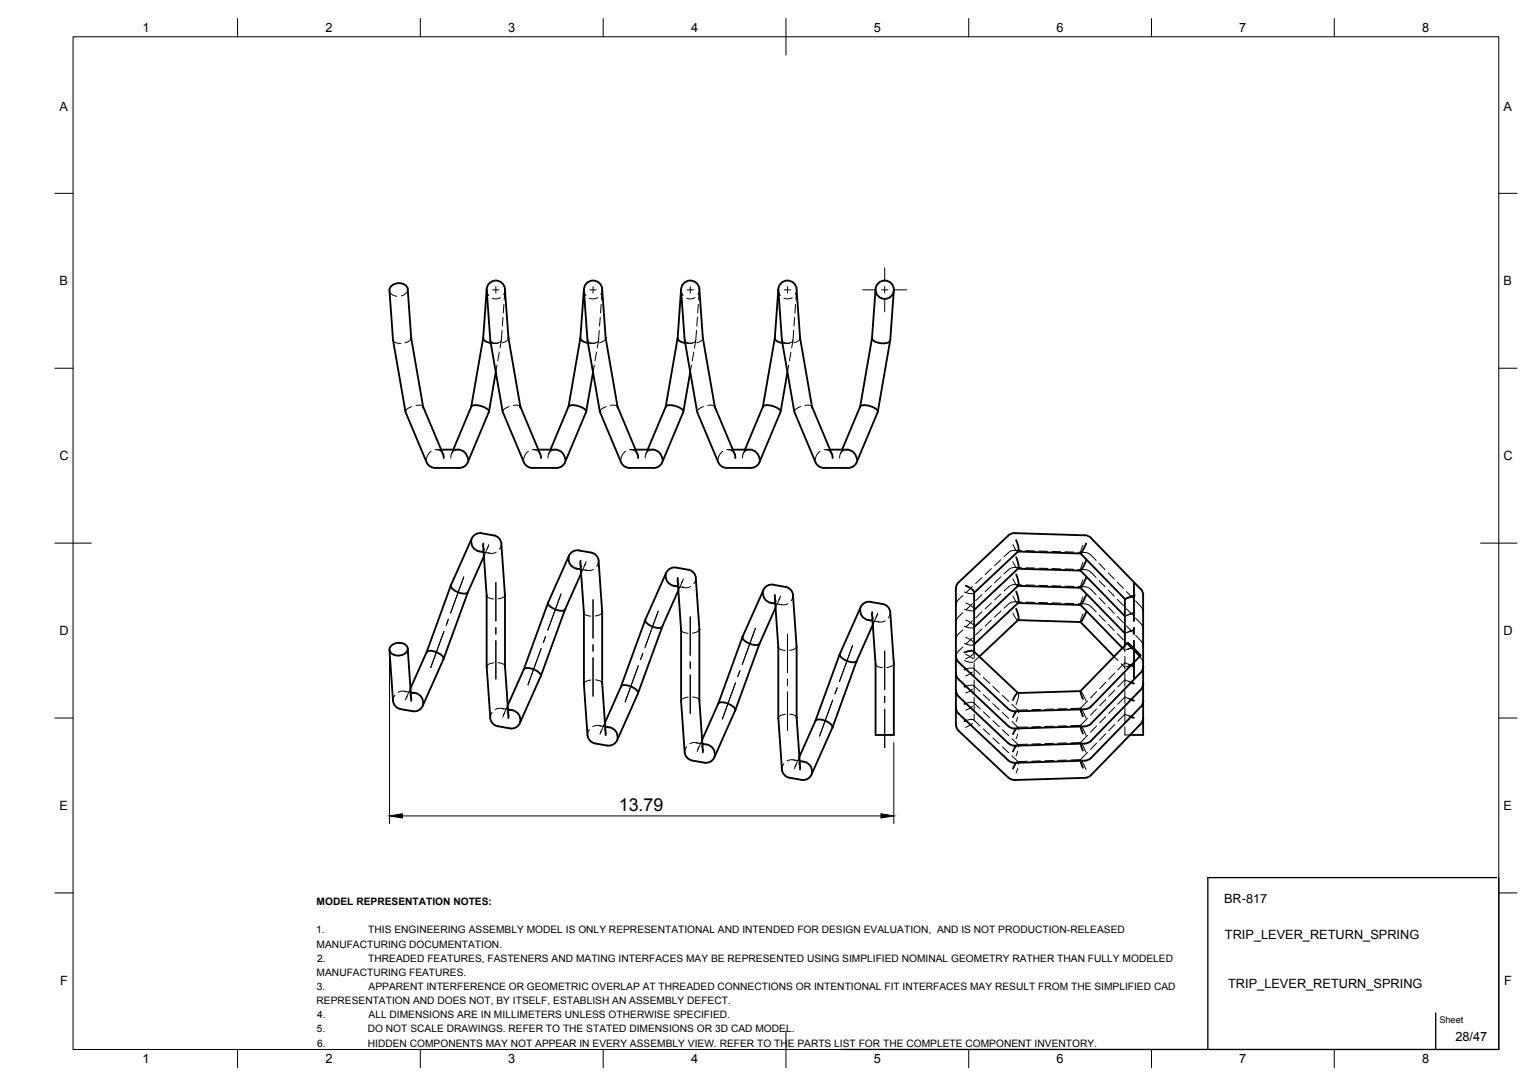
ISO-10303-21;
HEADER;
FILE_DESCRIPTION((''),'2;1');
FILE_NAME('TRIP_LEVER_RETURN_SPRING.step','2026-10-01T22:07:29-07:00',(''),(''),'','','');
FILE_SCHEMA (('AUTOMOTIVE_DESIGN { 1 0 10303 214 3 1 1 }'));
ENDSEC;
DATA;
#10=MECHANICAL_DESIGN_GEOMETRIC_PRESENTATION_REPRESENTATION('',(#560),#15484);
#15=ELLIPSE('',#9204,0.0269900326446259,0.025) ;
#16=ELLIPSE('',#9205,0.0269900326446259,0.025) ;
#17=ELLIPSE('',#9206,0.0269900326446259,0.025) ;
#18=ELLIPSE('',#9209,0.026990032644626,0.025) ;
#19=ELLIPSE('',#9210,0.026990032644626,0.025) ;
#20=ELLIPSE('',#9212,0.026990032644626,0.025) ;
#21=ELLIPSE('',#9214,0.026990032644626,0.025) ;
#22=ELLIPSE('',#9216,0.0269900326446258,0.025) ;
#23=ELLIPSE('',#9218,0.0269900326446259,0.025) ;
#24=ELLIPSE('',#9219,0.0269900326446259,0.025) ;
#25=ELLIPSE('',#9221,0.026990032644626,0.025) ;
#26=ELLIPSE('',#9222,0.026990032644626,0.025) ;
#27=ELLIPSE('',#9223,0.026990032644626,0.025) ;
#28=ELLIPSE('',#9225,0.026990032644626,0.025) ;
#29=ELLIPSE('',#9226,0.026990032644626,0.025) ;
#30=ELLIPSE('',#9228,0.0269900326446259,0.025) ;
#31=ELLIPSE('',#9229,0.0269900326446259,0.025) ;
#32=ELLIPSE('',#9230,0.0269900326446259,0.025) ;
#33=ELLIPSE('',#9232,0.026990032644626,0.025) ;
#34=ELLIPSE('',#9233,0.026990032644626,0.025) ;
#35=ELLIPSE('',#9235,0.0269900326446259,0.025) ;
#36=ELLIPSE('',#9237,0.026990032644626,0.025) ;
#37=ELLIPSE('',#9239,0.026990032644626,0.025) ;
#38=ELLIPSE('',#9241,0.0269900326446259,0.025) ;
#39=ELLIPSE('',#9242,0.0269900326446259,0.025) ;
#40=ELLIPSE('',#9244,0.026990032644626,0.025) ;
#41=ELLIPSE('',#9245,0.026990032644626,0.025) ;
#42=ELLIPSE('',#9246,0.026990032644626,0.025) ;
#43=ELLIPSE('',#9248,0.0269900326446259,0.025) ;
#44=ELLIPSE('',#9249,0.0269900326446259,0.025) ;
#45=ELLIPSE('',#9251,0.0269900326446258,0.025) ;
#46=ELLIPSE('',#9252,0.0269900326446258,0.025) ;
#47=ELLIPSE('',#9253,0.0269900326446258,0.025) ;
#48=ELLIPSE('',#9255,0.0269900326446259,0.025) ;
#49=ELLIPSE('',#9256,0.0269900326446259,0.025) ;
#50=ELLIPSE('',#9258,0.0269900326446259,0.025) ;
#51=ELLIPSE('',#9260,0.026990032644626,0.025) ;
#52=ELLIPSE('',#9262,0.0269900326446259,0.025) ;
#53=ELLIPSE('',#9264,0.026990032644626,0.025) ;
#54=ELLIPSE('',#9265,0.026990032644626,0.025) ;
#55=ELLIPSE('',#9267,0.026990032644626,0.025) ;
#56=ELLIPSE('',#9268,0.026990032644626,0.025) ;
#57=ELLIPSE('',#9269,0.026990032644626,0.025) ;
#58=ELLIPSE('',#9271,0.026990032644626,0.025) ;
#59=ELLIPSE('',#9272,0.026990032644626,0.025) ;
#60=ELLIPSE('',#9274,0.0269900326446259,0.025) ;
#61=ELLIPSE('',#9275,0.0269900326446259,0.025) ;
#62=ELLIPSE('',#9276,0.0269900326446259,0.025) ;
#63=ELLIPSE('',#9278,0.0269900326446259,0.025) ;
#64=ELLIPSE('',#9279,0.0269900326446259,0.025) ;
#65=ELLIPSE('',#9281,0.0269900326446259,0.025) ;
#66=ELLIPSE('',#9283,0.026990032644626,0.025) ;
#67=ELLIPSE('',#9285,0.0269900326446259,0.025) ;
#68=ELLIPSE('',#9287,0.0269900326446259,0.025) ;
#69=ELLIPSE('',#9288,0.0269900326446259,0.025) ;
#70=ELLIPSE('',#9290,0.026990032644626,0.025) ;
#71=ELLIPSE('',#9291,0.026990032644626,0.025) ;
#72=ELLIPSE('',#9292,0.026990032644626,0.025) ;
#73=ELLIPSE('',#9294,0.0269900326446259,0.025) ;
#74=ELLIPSE('',#9295,0.0269900326446259,0.025) ;
#75=ELLIPSE('',#9297,0.0269900326446259,0.025) ;
#76=ELLIPSE('',#9298,0.0269900326446259,0.025) ;
#77=ELLIPSE('',#9299,0.0269900326446259,0.025) ;
#78=ELLIPSE('',#9301,0.0269900326446259,0.025) ;
#79=ELLIPSE('',#9302,0.0269900326446259,0.025) ;
#80=ELLIPSE('',#9304,0.0269900326446259,0.025) ;
#81=ELLIPSE('',#9306,0.026990032644626,0.025) ;
#82=ELLIPSE('',#9308,0.0269900326446259,0.025) ;
#83=ELLIPSE('',#9310,0.026990032644626,0.025) ;
#84=ELLIPSE('',#9311,0.026990032644626,0.025) ;
#85=ELLIPSE('',#9313,0.026990032644626,0.025) ;
#86=ELLIPSE('',#9314,0.026990032644626,0.025) ;
#87=ELLIPSE('',#9315,0.026990032644626,0.025) ;
#198=SPHERICAL_SURFACE('',#9045,0.025) ;
#199=SPHERICAL_SURFACE('',#9048,0.025) ;
#200=SPHERICAL_SURFACE('',#9052,0.025) ;
#201=SPHERICAL_SURFACE('',#9057,0.025) ;
#202=SPHERICAL_SURFACE('',#9062,0.025) ;
#203=SPHERICAL_SURFACE('',#9067,0.025) ;
#204=SPHERICAL_SURFACE('',#9071,0.025) ;
#205=SPHERICAL_SURFACE('',#9074,0.025) ;
#206=SPHERICAL_SURFACE('',#9077,0.025) ;
#207=SPHERICAL_SURFACE('',#9080,0.025) ;
#208=SPHERICAL_SURFACE('',#9084,0.025) ;
#209=SPHERICAL_SURFACE('',#9089,0.025) ;
#210=SPHERICAL_SURFACE('',#9094,0.025) ;
#211=SPHERICAL_SURFACE('',#9099,0.025) ;
#212=SPHERICAL_SURFACE('',#9103,0.025) ;
#213=SPHERICAL_SURFACE('',#9106,0.025) ;
#214=SPHERICAL_SURFACE('',#9109,0.025) ;
#215=SPHERICAL_SURFACE('',#9112,0.025) ;
#216=SPHERICAL_SURFACE('',#9116,0.025) ;
#217=SPHERICAL_SURFACE('',#9121,0.025) ;
#218=SPHERICAL_SURFACE('',#9126,0.025) ;
#219=SPHERICAL_SURFACE('',#9131,0.025) ;
#220=SPHERICAL_SURFACE('',#9135,0.025) ;
#221=SPHERICAL_SURFACE('',#9138,0.025) ;
#222=SPHERICAL_SURFACE('',#9141,0.025) ;
#223=SPHERICAL_SURFACE('',#9144,0.025) ;
#224=SPHERICAL_SURFACE('',#9148,0.025) ;
#225=SPHERICAL_SURFACE('',#9153,0.025) ;
#226=SPHERICAL_SURFACE('',#9158,0.025) ;
#227=SPHERICAL_SURFACE('',#9163,0.025) ;
#228=SPHERICAL_SURFACE('',#9167,0.025) ;
#229=SPHERICAL_SURFACE('',#9170,0.025) ;
#230=SPHERICAL_SURFACE('',#9173,0.025) ;
#231=SPHERICAL_SURFACE('',#9176,0.025) ;
#232=SPHERICAL_SURFACE('',#9180,0.025) ;
#233=SPHERICAL_SURFACE('',#9185,0.025) ;
#234=SPHERICAL_SURFACE('',#9190,0.025) ;
#235=SPHERICAL_SURFACE('',#9195,0.025) ;
#236=SPHERICAL_SURFACE('',#9199,0.025) ;
#490=SHAPE_REPRESENTATION_RELATIONSHIP('SRR','None',#15640,#525) ;
#525=ADVANCED_BREP_SHAPE_REPRESENTATION('',(#601),#15464) ;
#560=STYLED_ITEM('',(#15832),#601) ;
#601=MANIFOLD_SOLID_BREP('TRIP_LEVER_RETURN_SPRING',#8271) ;
#688=CYLINDRICAL_SURFACE('',#9202,0.025) ;
#689=CYLINDRICAL_SURFACE('',#9208,0.025) ;
#690=CYLINDRICAL_SURFACE('',#9211,0.025) ;
#691=CYLINDRICAL_SURFACE('',#9213,0.025) ;
#692=CYLINDRICAL_SURFACE('',#9215,0.025) ;
#693=CYLINDRICAL_SURFACE('',#9217,0.025) ;
#694=CYLINDRICAL_SURFACE('',#9220,0.025) ;
#695=CYLINDRICAL_SURFACE('',#9224,0.025) ;
#696=CYLINDRICAL_SURFACE('',#9227,0.025) ;
#697=CYLINDRICAL_SURFACE('',#9231,0.025) ;
#698=CYLINDRICAL_SURFACE('',#9234,0.025) ;
#699=CYLINDRICAL_SURFACE('',#9236,0.025) ;
#700=CYLINDRICAL_SURFACE('',#9238,0.025) ;
#701=CYLINDRICAL_SURFACE('',#9240,0.025) ;
#702=CYLINDRICAL_SURFACE('',#9243,0.025) ;
#703=CYLINDRICAL_SURFACE('',#9247,0.025) ;
#704=CYLINDRICAL_SURFACE('',#9250,0.025) ;
#705=CYLINDRICAL_SURFACE('',#9254,0.025) ;
#706=CYLINDRICAL_SURFACE('',#9257,0.025) ;
#707=CYLINDRICAL_SURFACE('',#9259,0.025) ;
#708=CYLINDRICAL_SURFACE('',#9261,0.025) ;
#709=CYLINDRICAL_SURFACE('',#9263,0.025) ;
#710=CYLINDRICAL_SURFACE('',#9266,0.025) ;
#711=CYLINDRICAL_SURFACE('',#9270,0.025) ;
#712=CYLINDRICAL_SURFACE('',#9273,0.025) ;
#713=CYLINDRICAL_SURFACE('',#9277,0.025) ;
#714=CYLINDRICAL_SURFACE('',#9280,0.025) ;
#715=CYLINDRICAL_SURFACE('',#9282,0.025) ;
#716=CYLINDRICAL_SURFACE('',#9284,0.025) ;
#717=CYLINDRICAL_SURFACE('',#9286,0.025) ;
#718=CYLINDRICAL_SURFACE('',#9289,0.025) ;
#719=CYLINDRICAL_SURFACE('',#9293,0.025) ;
#720=CYLINDRICAL_SURFACE('',#9296,0.025) ;
#721=CYLINDRICAL_SURFACE('',#9300,0.025) ;
#722=CYLINDRICAL_SURFACE('',#9303,0.025) ;
#723=CYLINDRICAL_SURFACE('',#9305,0.025) ;
#724=CYLINDRICAL_SURFACE('',#9307,0.025) ;
#725=CYLINDRICAL_SURFACE('',#9309,0.025) ;
#726=CYLINDRICAL_SURFACE('',#9312,0.025) ;
#727=CYLINDRICAL_SURFACE('',#9316,0.025) ;
#1019=CIRCLE('',#9046,0.025) ;
#1020=CIRCLE('',#9047,0.025) ;
#1021=CIRCLE('',#9049,0.025) ;
#1022=CIRCLE('',#9050,0.025) ;
#1023=CIRCLE('',#9051,0.025) ;
#1024=CIRCLE('',#9053,0.025) ;
#1025=CIRCLE('',#9054,0.025) ;
#1026=CIRCLE('',#9055,0.025) ;
#1027=CIRCLE('',#9056,0.025) ;
#1028=CIRCLE('',#9058,0.025) ;
#1029=CIRCLE('',#9059,0.025) ;
#1030=CIRCLE('',#9060,0.025) ;
#1031=CIRCLE('',#9061,0.025) ;
#1032=CIRCLE('',#9063,0.025) ;
#1033=CIRCLE('',#9064,0.025) ;
#1034=CIRCLE('',#9065,0.025) ;
#1035=CIRCLE('',#9066,0.025) ;
#1036=CIRCLE('',#9068,0.025) ;
#1037=CIRCLE('',#9069,0.025) ;
#1038=CIRCLE('',#9070,0.025) ;
#1039=CIRCLE('',#9072,0.025) ;
#1040=CIRCLE('',#9073,0.025) ;
#1041=CIRCLE('',#9075,0.025) ;
#1042=CIRCLE('',#9076,0.025) ;
#1043=CIRCLE('',#9078,0.025) ;
#1044=CIRCLE('',#9079,0.025) ;
#1045=CIRCLE('',#9081,0.025) ;
#1046=CIRCLE('',#9082,0.025) ;
#1047=CIRCLE('',#9083,0.025) ;
#1048=CIRCLE('',#9085,0.025) ;
#1049=CIRCLE('',#9086,0.025) ;
#1050=CIRCLE('',#9087,0.025) ;
#1051=CIRCLE('',#9088,0.025) ;
#1052=CIRCLE('',#9090,0.025) ;
#1053=CIRCLE('',#9091,0.025) ;
#1054=CIRCLE('',#9092,0.025) ;
#1055=CIRCLE('',#9093,0.025) ;
#1056=CIRCLE('',#9095,0.025) ;
#1057=CIRCLE('',#9096,0.025) ;
#1058=CIRCLE('',#9097,0.025) ;
#1059=CIRCLE('',#9098,0.025) ;
#1060=CIRCLE('',#9100,0.025) ;
#1061=CIRCLE('',#9101,0.025) ;
#1062=CIRCLE('',#9102,0.025) ;
#1063=CIRCLE('',#9104,0.025) ;
#1064=CIRCLE('',#9105,0.025) ;
#1065=CIRCLE('',#9107,0.025) ;
#1066=CIRCLE('',#9108,0.025) ;
#1067=CIRCLE('',#9110,0.025) ;
#1068=CIRCLE('',#9111,0.025) ;
#1069=CIRCLE('',#9113,0.025) ;
#1070=CIRCLE('',#9114,0.025) ;
#1071=CIRCLE('',#9115,0.025) ;
#1072=CIRCLE('',#9117,0.025) ;
#1073=CIRCLE('',#9118,0.025) ;
#1074=CIRCLE('',#9119,0.025) ;
#1075=CIRCLE('',#9120,0.025) ;
#1076=CIRCLE('',#9122,0.025) ;
#1077=CIRCLE('',#9123,0.025) ;
#1078=CIRCLE('',#9124,0.025) ;
#1079=CIRCLE('',#9125,0.025) ;
#1080=CIRCLE('',#9127,0.025) ;
#1081=CIRCLE('',#9128,0.025) ;
#1082=CIRCLE('',#9129,0.025) ;
#1083=CIRCLE('',#9130,0.025) ;
#1084=CIRCLE('',#9132,0.025) ;
#1085=CIRCLE('',#9133,0.025) ;
#1086=CIRCLE('',#9134,0.025) ;
#1087=CIRCLE('',#9136,0.025) ;
#1088=CIRCLE('',#9137,0.025) ;
#1089=CIRCLE('',#9139,0.025) ;
#1090=CIRCLE('',#9140,0.025) ;
#1091=CIRCLE('',#9142,0.025) ;
#1092=CIRCLE('',#9143,0.025) ;
#1093=CIRCLE('',#9145,0.025) ;
#1094=CIRCLE('',#9146,0.025) ;
#1095=CIRCLE('',#9147,0.025) ;
#1096=CIRCLE('',#9149,0.025) ;
#1097=CIRCLE('',#9150,0.025) ;
#1098=CIRCLE('',#9151,0.025) ;
#1099=CIRCLE('',#9152,0.025) ;
#1100=CIRCLE('',#9154,0.025) ;
#1101=CIRCLE('',#9155,0.025) ;
#1102=CIRCLE('',#9156,0.025) ;
#1103=CIRCLE('',#9157,0.025) ;
#1104=CIRCLE('',#9159,0.025) ;
#1105=CIRCLE('',#9160,0.025) ;
#1106=CIRCLE('',#9161,0.025) ;
#1107=CIRCLE('',#9162,0.025) ;
#1108=CIRCLE('',#9164,0.025) ;
#1109=CIRCLE('',#9165,0.025) ;
#1110=CIRCLE('',#9166,0.025) ;
#1111=CIRCLE('',#9168,0.025) ;
#1112=CIRCLE('',#9169,0.025) ;
#1113=CIRCLE('',#9171,0.025) ;
#1114=CIRCLE('',#9172,0.025) ;
#1115=CIRCLE('',#9174,0.025) ;
#1116=CIRCLE('',#9175,0.025) ;
#1117=CIRCLE('',#9177,0.025) ;
#1118=CIRCLE('',#9178,0.025) ;
#1119=CIRCLE('',#9179,0.025) ;
#1120=CIRCLE('',#9181,0.025) ;
#1121=CIRCLE('',#9182,0.025) ;
#1122=CIRCLE('',#9183,0.025) ;
#1123=CIRCLE('',#9184,0.025) ;
#1124=CIRCLE('',#9186,0.025) ;
#1125=CIRCLE('',#9187,0.025) ;
#1126=CIRCLE('',#9188,0.025) ;
#1127=CIRCLE('',#9189,0.025) ;
#1128=CIRCLE('',#9191,0.025) ;
#1129=CIRCLE('',#9192,0.025) ;
#1130=CIRCLE('',#9193,0.025) ;
#1131=CIRCLE('',#9194,0.025) ;
#1132=CIRCLE('',#9196,0.025) ;
#1133=CIRCLE('',#9197,0.025) ;
#1134=CIRCLE('',#9198,0.025) ;
#1135=CIRCLE('',#9200,0.025) ;
#1136=CIRCLE('',#9201,0.025) ;
#1137=CIRCLE('',#9203,0.025) ;
#1138=CIRCLE('',#9317,0.025) ;
#1554=FACE_OUTER_BOUND('',#2115,.T.) ;
#1555=FACE_OUTER_BOUND('',#2116,.T.) ;
#1556=FACE_OUTER_BOUND('',#2117,.T.) ;
#1557=FACE_OUTER_BOUND('',#2118,.T.) ;
#1558=FACE_OUTER_BOUND('',#2119,.T.) ;
#1559=FACE_OUTER_BOUND('',#2120,.T.) ;
#1560=FACE_OUTER_BOUND('',#2121,.T.) ;
#1561=FACE_OUTER_BOUND('',#2122,.T.) ;
#1562=FACE_OUTER_BOUND('',#2123,.T.) ;
#1563=FACE_OUTER_BOUND('',#2124,.T.) ;
#1564=FACE_OUTER_BOUND('',#2125,.T.) ;
#1565=FACE_OUTER_BOUND('',#2126,.T.) ;
#1566=FACE_OUTER_BOUND('',#2127,.T.) ;
#1567=FACE_OUTER_BOUND('',#2128,.T.) ;
#1568=FACE_OUTER_BOUND('',#2129,.T.) ;
#1569=FACE_OUTER_BOUND('',#2130,.T.) ;
#1570=FACE_OUTER_BOUND('',#2131,.T.) ;
#1571=FACE_OUTER_BOUND('',#2132,.T.) ;
#1572=FACE_OUTER_BOUND('',#2133,.T.) ;
#1573=FACE_OUTER_BOUND('',#2134,.T.) ;
#1574=FACE_OUTER_BOUND('',#2135,.T.) ;
#1575=FACE_OUTER_BOUND('',#2136,.T.) ;
#1576=FACE_OUTER_BOUND('',#2137,.T.) ;
#1577=FACE_OUTER_BOUND('',#2138,.T.) ;
#1578=FACE_OUTER_BOUND('',#2139,.T.) ;
#1579=FACE_OUTER_BOUND('',#2140,.T.) ;
#1580=FACE_OUTER_BOUND('',#2141,.T.) ;
#1581=FACE_OUTER_BOUND('',#2142,.T.) ;
#1582=FACE_OUTER_BOUND('',#2143,.T.) ;
#1583=FACE_OUTER_BOUND('',#2144,.T.) ;
#1584=FACE_OUTER_BOUND('',#2145,.T.) ;
#1585=FACE_OUTER_BOUND('',#2146,.T.) ;
#1586=FACE_OUTER_BOUND('',#2147,.T.) ;
#1587=FACE_OUTER_BOUND('',#2148,.T.) ;
#1588=FACE_OUTER_BOUND('',#2149,.T.) ;
#1589=FACE_OUTER_BOUND('',#2150,.T.) ;
#1590=FACE_OUTER_BOUND('',#2151,.T.) ;
#1591=FACE_OUTER_BOUND('',#2152,.T.) ;
#1592=FACE_OUTER_BOUND('',#2153,.T.) ;
#1593=FACE_OUTER_BOUND('',#2154,.T.) ;
#1594=FACE_OUTER_BOUND('',#2155,.T.) ;
#1595=FACE_OUTER_BOUND('',#2156,.T.) ;
#1596=FACE_OUTER_BOUND('',#2157,.T.) ;
#1597=FACE_OUTER_BOUND('',#2158,.T.) ;
#1598=FACE_OUTER_BOUND('',#2159,.T.) ;
#1599=FACE_OUTER_BOUND('',#2160,.T.) ;
#1600=FACE_OUTER_BOUND('',#2161,.T.) ;
#1601=FACE_OUTER_BOUND('',#2162,.T.) ;
#1602=FACE_OUTER_BOUND('',#2163,.T.) ;
#1603=FACE_OUTER_BOUND('',#2164,.T.) ;
#1604=FACE_OUTER_BOUND('',#2165,.T.) ;
#1605=FACE_OUTER_BOUND('',#2166,.T.) ;
#1606=FACE_OUTER_BOUND('',#2167,.T.) ;
#1607=FACE_OUTER_BOUND('',#2168,.T.) ;
#1608=FACE_OUTER_BOUND('',#2169,.T.) ;
#1609=FACE_OUTER_BOUND('',#2170,.T.) ;
#1610=FACE_OUTER_BOUND('',#2171,.T.) ;
#1611=FACE_OUTER_BOUND('',#2172,.T.) ;
#1612=FACE_OUTER_BOUND('',#2173,.T.) ;
#1613=FACE_OUTER_BOUND('',#2174,.T.) ;
#1614=FACE_OUTER_BOUND('',#2175,.T.) ;
#1615=FACE_OUTER_BOUND('',#2176,.T.) ;
#1616=FACE_OUTER_BOUND('',#2177,.T.) ;
#1617=FACE_OUTER_BOUND('',#2178,.T.) ;
#1618=FACE_OUTER_BOUND('',#2179,.T.) ;
#1619=FACE_OUTER_BOUND('',#2180,.T.) ;
#1620=FACE_OUTER_BOUND('',#2181,.T.) ;
#1621=FACE_OUTER_BOUND('',#2182,.T.) ;
#1622=FACE_OUTER_BOUND('',#2183,.T.) ;
#1623=FACE_OUTER_BOUND('',#2184,.T.) ;
#1624=FACE_OUTER_BOUND('',#2185,.T.) ;
#1625=FACE_OUTER_BOUND('',#2186,.T.) ;
#1626=FACE_OUTER_BOUND('',#2187,.T.) ;
#1627=FACE_OUTER_BOUND('',#2188,.T.) ;
#1628=FACE_OUTER_BOUND('',#2189,.T.) ;
#1629=FACE_OUTER_BOUND('',#2190,.T.) ;
#1630=FACE_OUTER_BOUND('',#2191,.T.) ;
#1631=FACE_OUTER_BOUND('',#2192,.T.) ;
#1632=FACE_OUTER_BOUND('',#2193,.T.) ;
#1633=FACE_OUTER_BOUND('',#2194,.T.) ;
#1634=FACE_OUTER_BOUND('',#2195,.T.) ;
#2115=EDGE_LOOP('',(#6027,#6028)) ;
#2116=EDGE_LOOP('',(#6029,#6030,#6031)) ;
#2117=EDGE_LOOP('',(#6032,#6033,#6034,#6035)) ;
#2118=EDGE_LOOP('',(#6036,#6037,#6038,#6039)) ;
#2119=EDGE_LOOP('',(#6040,#6041,#6042,#6043)) ;
#2120=EDGE_LOOP('',(#6044,#6045,#6046)) ;
#2121=EDGE_LOOP('',(#6047,#6048)) ;
#2122=EDGE_LOOP('',(#6049,#6050)) ;
#2123=EDGE_LOOP('',(#6051,#6052)) ;
#2124=EDGE_LOOP('',(#6053,#6054,#6055)) ;
#2125=EDGE_LOOP('',(#6056,#6057,#6058,#6059)) ;
#2126=EDGE_LOOP('',(#6060,#6061,#6062,#6063)) ;
#2127=EDGE_LOOP('',(#6064,#6065,#6066,#6067)) ;
#2128=EDGE_LOOP('',(#6068,#6069,#6070)) ;
#2129=EDGE_LOOP('',(#6071,#6072)) ;
#2130=EDGE_LOOP('',(#6073,#6074)) ;
#2131=EDGE_LOOP('',(#6075,#6076)) ;
#2132=EDGE_LOOP('',(#6077,#6078,#6079)) ;
#2133=EDGE_LOOP('',(#6080,#6081,#6082,#6083)) ;
#2134=EDGE_LOOP('',(#6084,#6085,#6086,#6087)) ;
#2135=EDGE_LOOP('',(#6088,#6089,#6090,#6091)) ;
#2136=EDGE_LOOP('',(#6092,#6093,#6094)) ;
#2137=EDGE_LOOP('',(#6095,#6096)) ;
#2138=EDGE_LOOP('',(#6097,#6098)) ;
#2139=EDGE_LOOP('',(#6099,#6100)) ;
#2140=EDGE_LOOP('',(#6101,#6102,#6103)) ;
#2141=EDGE_LOOP('',(#6104,#6105,#6106,#6107)) ;
#2142=EDGE_LOOP('',(#6108,#6109,#6110,#6111)) ;
#2143=EDGE_LOOP('',(#6112,#6113,#6114,#6115)) ;
#2144=EDGE_LOOP('',(#6116,#6117,#6118)) ;
#2145=EDGE_LOOP('',(#6119,#6120)) ;
#2146=EDGE_LOOP('',(#6121,#6122)) ;
#2147=EDGE_LOOP('',(#6123,#6124)) ;
#2148=EDGE_LOOP('',(#6125,#6126,#6127)) ;
#2149=EDGE_LOOP('',(#6128,#6129,#6130,#6131)) ;
#2150=EDGE_LOOP('',(#6132,#6133,#6134,#6135)) ;
#2151=EDGE_LOOP('',(#6136,#6137,#6138,#6139)) ;
#2152=EDGE_LOOP('',(#6140,#6141,#6142)) ;
#2153=EDGE_LOOP('',(#6143,#6144)) ;
#2154=EDGE_LOOP('',(#6145,#6146,#6147,#6148,#6149,#6150,#6151)) ;
#2155=EDGE_LOOP('',(#6152)) ;
#2156=EDGE_LOOP('',(#6153,#6154,#6155,#6156,#6157,#6158,#6159,#6160,#6161)) ;
#2157=EDGE_LOOP('',(#6162,#6163,#6164,#6165,#6166,#6167,#6168,#6169,#6170)) ;
#2158=EDGE_LOOP('',(#6171,#6172,#6173,#6174,#6175,#6176,#6177,#6178)) ;
#2159=EDGE_LOOP('',(#6179,#6180,#6181,#6182,#6183,#6184,#6185,#6186)) ;
#2160=EDGE_LOOP('',(#6187,#6188,#6189,#6190,#6191,#6192,#6193,#6194,#6195)) ;
#2161=EDGE_LOOP('',(#6196,#6197,#6198,#6199,#6200,#6201,#6202,#6203,#6204)) ;
#2162=EDGE_LOOP('',(#6205,#6206,#6207,#6208,#6209,#6210,#6211,#6212,#6213)) ;
#2163=EDGE_LOOP('',(#6214,#6215,#6216,#6217,#6218,#6219,#6220,#6221,#6222)) ;
#2164=EDGE_LOOP('',(#6223,#6224,#6225,#6226,#6227,#6228,#6229,#6230,#6231)) ;
#2165=EDGE_LOOP('',(#6232,#6233,#6234,#6235,#6236,#6237,#6238,#6239,#6240)) ;
#2166=EDGE_LOOP('',(#6241,#6242,#6243,#6244,#6245,#6246,#6247,#6248)) ;
#2167=EDGE_LOOP('',(#6249,#6250,#6251,#6252,#6253,#6254,#6255,#6256)) ;
#2168=EDGE_LOOP('',(#6257,#6258,#6259,#6260,#6261,#6262,#6263,#6264,#6265)) ;
#2169=EDGE_LOOP('',(#6266,#6267,#6268,#6269,#6270,#6271,#6272,#6273,#6274)) ;
#2170=EDGE_LOOP('',(#6275,#6276,#6277,#6278,#6279,#6280,#6281,#6282,#6283)) ;
#2171=EDGE_LOOP('',(#6284,#6285,#6286,#6287,#6288,#6289,#6290,#6291,#6292)) ;
#2172=EDGE_LOOP('',(#6293,#6294,#6295,#6296,#6297,#6298,#6299,#6300,#6301)) ;
#2173=EDGE_LOOP('',(#6302,#6303,#6304,#6305,#6306,#6307,#6308,#6309,#6310)) ;
#2174=EDGE_LOOP('',(#6311,#6312,#6313,#6314,#6315,#6316,#6317,#6318)) ;
#2175=EDGE_LOOP('',(#6319,#6320,#6321,#6322,#6323,#6324,#6325,#6326)) ;
#2176=EDGE_LOOP('',(#6327,#6328,#6329,#6330,#6331,#6332,#6333,#6334,#6335)) ;
#2177=EDGE_LOOP('',(#6336,#6337,#6338,#6339,#6340,#6341,#6342,#6343,#6344)) ;
#2178=EDGE_LOOP('',(#6345,#6346,#6347,#6348,#6349,#6350,#6351,#6352,#6353)) ;
#2179=EDGE_LOOP('',(#6354,#6355,#6356,#6357,#6358,#6359,#6360,#6361,#6362)) ;
#2180=EDGE_LOOP('',(#6363,#6364,#6365,#6366,#6367,#6368,#6369,#6370,#6371)) ;
#2181=EDGE_LOOP('',(#6372,#6373,#6374,#6375,#6376,#6377,#6378,#6379,#6380)) ;
#2182=EDGE_LOOP('',(#6381,#6382,#6383,#6384,#6385,#6386,#6387,#6388)) ;
#2183=EDGE_LOOP('',(#6389,#6390,#6391,#6392,#6393,#6394,#6395,#6396)) ;
#2184=EDGE_LOOP('',(#6397,#6398,#6399,#6400,#6401,#6402,#6403,#6404,#6405)) ;
#2185=EDGE_LOOP('',(#6406,#6407,#6408,#6409,#6410,#6411,#6412,#6413,#6414)) ;
#2186=EDGE_LOOP('',(#6415,#6416,#6417,#6418,#6419,#6420,#6421,#6422,#6423)) ;
#2187=EDGE_LOOP('',(#6424,#6425,#6426,#6427,#6428,#6429,#6430,#6431,#6432)) ;
#2188=EDGE_LOOP('',(#6433,#6434,#6435,#6436,#6437,#6438,#6439,#6440,#6441)) ;
#2189=EDGE_LOOP('',(#6442,#6443,#6444,#6445,#6446,#6447,#6448,#6449,#6450)) ;
#2190=EDGE_LOOP('',(#6451,#6452,#6453,#6454,#6455,#6456,#6457,#6458)) ;
#2191=EDGE_LOOP('',(#6459,#6460,#6461,#6462,#6463,#6464,#6465,#6466)) ;
#2192=EDGE_LOOP('',(#6467,#6468,#6469,#6470,#6471,#6472,#6473,#6474,#6475)) ;
#2193=EDGE_LOOP('',(#6476,#6477,#6478,#6479,#6480,#6481,#6482,#6483,#6484)) ;
#2194=EDGE_LOOP('',(#6485,#6486,#6487,#6488,#6489,#6490,#6491)) ;
#2195=EDGE_LOOP('',(#6492)) ;
#2679=LINE('',#14063,#3153) ;
#2680=LINE('',#14071,#3154) ;
#2681=LINE('',#14075,#3155) ;
#2682=LINE('',#14078,#3156) ;
#2683=LINE('',#14081,#3157) ;
#2684=LINE('',#14084,#3158) ;
#2685=LINE('',#14090,#3159) ;
#2686=LINE('',#14097,#3160) ;
#2687=LINE('',#14102,#3161) ;
#2688=LINE('',#14109,#3162) ;
#2689=LINE('',#14113,#3163) ;
#2690=LINE('',#14116,#3164) ;
#2691=LINE('',#14119,#3165) ;
#2692=LINE('',#14122,#3166) ;
#2693=LINE('',#14128,#3167) ;
#2694=LINE('',#14135,#3168) ;
#2695=LINE('',#14140,#3169) ;
#2696=LINE('',#14147,#3170) ;
#2697=LINE('',#14151,#3171) ;
#2698=LINE('',#14154,#3172) ;
#2699=LINE('',#14157,#3173) ;
#2700=LINE('',#14160,#3174) ;
#2701=LINE('',#14166,#3175) ;
#2702=LINE('',#14173,#3176) ;
#2703=LINE('',#14178,#3177) ;
#2704=LINE('',#14185,#3178) ;
#2705=LINE('',#14189,#3179) ;
#2706=LINE('',#14192,#3180) ;
#2707=LINE('',#14195,#3181) ;
#2708=LINE('',#14198,#3182) ;
#2709=LINE('',#14204,#3183) ;
#2710=LINE('',#14211,#3184) ;
#2711=LINE('',#14216,#3185) ;
#2712=LINE('',#14223,#3186) ;
#2713=LINE('',#14227,#3187) ;
#2714=LINE('',#14230,#3188) ;
#2715=LINE('',#14233,#3189) ;
#2716=LINE('',#14236,#3190) ;
#2717=LINE('',#14242,#3191) ;
#2718=LINE('',#14249,#3192) ;
#3153=VECTOR('',#11208,0.025) ;
#3154=VECTOR('',#11219,0.025) ;
#3155=VECTOR('',#11226,0.025) ;
#3156=VECTOR('',#11231,0.025) ;
#3157=VECTOR('',#11236,0.025) ;
#3158=VECTOR('',#11241,0.025) ;
#3159=VECTOR('',#11248,0.025) ;
#3160=VECTOR('',#11257,0.025) ;
#3161=VECTOR('',#11264,0.025) ;
#3162=VECTOR('',#11273,0.025) ;
#3163=VECTOR('',#11280,0.025) ;
#3164=VECTOR('',#11285,0.025) ;
#3165=VECTOR('',#11290,0.025) ;
#3166=VECTOR('',#11295,0.025) ;
#3167=VECTOR('',#11302,0.025) ;
#3168=VECTOR('',#11311,0.025) ;
#3169=VECTOR('',#11318,0.025) ;
#3170=VECTOR('',#11327,0.025) ;
#3171=VECTOR('',#11334,0.025) ;
#3172=VECTOR('',#11339,0.025) ;
#3173=VECTOR('',#11344,0.025) ;
#3174=VECTOR('',#11349,0.025) ;
#3175=VECTOR('',#11356,0.025) ;
#3176=VECTOR('',#11365,0.025) ;
#3177=VECTOR('',#11372,0.025) ;
#3178=VECTOR('',#11381,0.025) ;
#3179=VECTOR('',#11388,0.025) ;
#3180=VECTOR('',#11393,0.025) ;
#3181=VECTOR('',#11398,0.025) ;
#3182=VECTOR('',#11403,0.025) ;
#3183=VECTOR('',#11410,0.025) ;
#3184=VECTOR('',#11419,0.025) ;
#3185=VECTOR('',#11426,0.025) ;
#3186=VECTOR('',#11435,0.025) ;
#3187=VECTOR('',#11442,0.025) ;
#3188=VECTOR('',#11447,0.025) ;
#3189=VECTOR('',#11452,0.025) ;
#3190=VECTOR('',#11457,0.025) ;
#3191=VECTOR('',#11464,0.025) ;
#3192=VECTOR('',#11473,0.025) ;
#3641=VERTEX_POINT('',#13785) ;
#3642=VERTEX_POINT('',#13786) ;
#3643=VERTEX_POINT('',#13790) ;
#3644=VERTEX_POINT('',#13791) ;
#3645=VERTEX_POINT('',#13793) ;
#3646=VERTEX_POINT('',#13797) ;
#3647=VERTEX_POINT('',#13798) ;
#3648=VERTEX_POINT('',#13800) ;
#3649=VERTEX_POINT('',#13802) ;
#3650=VERTEX_POINT('',#13806) ;
#3651=VERTEX_POINT('',#13807) ;
#3652=VERTEX_POINT('',#13809) ;
#3653=VERTEX_POINT('',#13811) ;
#3654=VERTEX_POINT('',#13815) ;
#3655=VERTEX_POINT('',#13816) ;
#3656=VERTEX_POINT('',#13818) ;
#3657=VERTEX_POINT('',#13820) ;
#3658=VERTEX_POINT('',#13824) ;
#3659=VERTEX_POINT('',#13825) ;
#3660=VERTEX_POINT('',#13827) ;
#3661=VERTEX_POINT('',#13831) ;
#3662=VERTEX_POINT('',#13832) ;
#3663=VERTEX_POINT('',#13836) ;
#3664=VERTEX_POINT('',#13837) ;
#3665=VERTEX_POINT('',#13841) ;
#3666=VERTEX_POINT('',#13842) ;
#3667=VERTEX_POINT('',#13846) ;
#3668=VERTEX_POINT('',#13847) ;
#3669=VERTEX_POINT('',#13849) ;
#3670=VERTEX_POINT('',#13853) ;
#3671=VERTEX_POINT('',#13854) ;
#3672=VERTEX_POINT('',#13856) ;
#3673=VERTEX_POINT('',#13858) ;
#3674=VERTEX_POINT('',#13862) ;
#3675=VERTEX_POINT('',#13863) ;
#3676=VERTEX_POINT('',#13865) ;
#3677=VERTEX_POINT('',#13867) ;
#3678=VERTEX_POINT('',#13871) ;
#3679=VERTEX_POINT('',#13872) ;
#3680=VERTEX_POINT('',#13874) ;
#3681=VERTEX_POINT('',#13876) ;
#3682=VERTEX_POINT('',#13880) ;
#3683=VERTEX_POINT('',#13881) ;
#3684=VERTEX_POINT('',#13883) ;
#3685=VERTEX_POINT('',#13887) ;
#3686=VERTEX_POINT('',#13888) ;
#3687=VERTEX_POINT('',#13892) ;
#3688=VERTEX_POINT('',#13893) ;
#3689=VERTEX_POINT('',#13897) ;
#3690=VERTEX_POINT('',#13898) ;
#3691=VERTEX_POINT('',#13902) ;
#3692=VERTEX_POINT('',#13903) ;
#3693=VERTEX_POINT('',#13905) ;
#3694=VERTEX_POINT('',#13909) ;
#3695=VERTEX_POINT('',#13910) ;
#3696=VERTEX_POINT('',#13912) ;
#3697=VERTEX_POINT('',#13914) ;
#3698=VERTEX_POINT('',#13918) ;
#3699=VERTEX_POINT('',#13919) ;
#3700=VERTEX_POINT('',#13921) ;
#3701=VERTEX_POINT('',#13923) ;
#3702=VERTEX_POINT('',#13927) ;
#3703=VERTEX_POINT('',#13928) ;
#3704=VERTEX_POINT('',#13930) ;
#3705=VERTEX_POINT('',#13932) ;
#3706=VERTEX_POINT('',#13936) ;
#3707=VERTEX_POINT('',#13937) ;
#3708=VERTEX_POINT('',#13939) ;
#3709=VERTEX_POINT('',#13943) ;
#3710=VERTEX_POINT('',#13944) ;
#3711=VERTEX_POINT('',#13948) ;
#3712=VERTEX_POINT('',#13949) ;
#3713=VERTEX_POINT('',#13953) ;
#3714=VERTEX_POINT('',#13954) ;
#3715=VERTEX_POINT('',#13958) ;
#3716=VERTEX_POINT('',#13959) ;
#3717=VERTEX_POINT('',#13961) ;
#3718=VERTEX_POINT('',#13965) ;
#3719=VERTEX_POINT('',#13966) ;
#3720=VERTEX_POINT('',#13968) ;
#3721=VERTEX_POINT('',#13970) ;
#3722=VERTEX_POINT('',#13974) ;
#3723=VERTEX_POINT('',#13975) ;
#3724=VERTEX_POINT('',#13977) ;
#3725=VERTEX_POINT('',#13979) ;
#3726=VERTEX_POINT('',#13983) ;
#3727=VERTEX_POINT('',#13984) ;
#3728=VERTEX_POINT('',#13986) ;
#3729=VERTEX_POINT('',#13988) ;
#3730=VERTEX_POINT('',#13992) ;
#3731=VERTEX_POINT('',#13993) ;
#3732=VERTEX_POINT('',#13995) ;
#3733=VERTEX_POINT('',#13999) ;
#3734=VERTEX_POINT('',#14000) ;
#3735=VERTEX_POINT('',#14004) ;
#3736=VERTEX_POINT('',#14005) ;
#3737=VERTEX_POINT('',#14009) ;
#3738=VERTEX_POINT('',#14010) ;
#3739=VERTEX_POINT('',#14014) ;
#3740=VERTEX_POINT('',#14015) ;
#3741=VERTEX_POINT('',#14017) ;
#3742=VERTEX_POINT('',#14021) ;
#3743=VERTEX_POINT('',#14022) ;
#3744=VERTEX_POINT('',#14024) ;
#3745=VERTEX_POINT('',#14026) ;
#3746=VERTEX_POINT('',#14030) ;
#3747=VERTEX_POINT('',#14031) ;
#3748=VERTEX_POINT('',#14033) ;
#3749=VERTEX_POINT('',#14035) ;
#3750=VERTEX_POINT('',#14039) ;
#3751=VERTEX_POINT('',#14040) ;
#3752=VERTEX_POINT('',#14042) ;
#3753=VERTEX_POINT('',#14044) ;
#3754=VERTEX_POINT('',#14048) ;
#3755=VERTEX_POINT('',#14049) ;
#3756=VERTEX_POINT('',#14051) ;
#3757=VERTEX_POINT('',#14055) ;
#3758=VERTEX_POINT('',#14056) ;
#3759=VERTEX_POINT('',#14060) ;
#3760=VERTEX_POINT('',#14062) ;
#3761=VERTEX_POINT('',#14064) ;
#3762=VERTEX_POINT('',#14070) ;
#3763=VERTEX_POINT('',#14085) ;
#3764=VERTEX_POINT('',#14089) ;
#3765=VERTEX_POINT('',#14091) ;
#3766=VERTEX_POINT('',#14096) ;
#3767=VERTEX_POINT('',#14101) ;
#3768=VERTEX_POINT('',#14103) ;
#3769=VERTEX_POINT('',#14108) ;
#3770=VERTEX_POINT('',#14123) ;
#3771=VERTEX_POINT('',#14127) ;
#3772=VERTEX_POINT('',#14129) ;
#3773=VERTEX_POINT('',#14134) ;
#3774=VERTEX_POINT('',#14139) ;
#3775=VERTEX_POINT('',#14141) ;
#3776=VERTEX_POINT('',#14146) ;
#3777=VERTEX_POINT('',#14161) ;
#3778=VERTEX_POINT('',#14165) ;
#3779=VERTEX_POINT('',#14167) ;
#3780=VERTEX_POINT('',#14172) ;
#3781=VERTEX_POINT('',#14177) ;
#3782=VERTEX_POINT('',#14179) ;
#3783=VERTEX_POINT('',#14184) ;
#3784=VERTEX_POINT('',#14199) ;
#3785=VERTEX_POINT('',#14203) ;
#3786=VERTEX_POINT('',#14205) ;
#3787=VERTEX_POINT('',#14210) ;
#3788=VERTEX_POINT('',#14215) ;
#3789=VERTEX_POINT('',#14217) ;
#3790=VERTEX_POINT('',#14222) ;
#3791=VERTEX_POINT('',#14237) ;
#3792=VERTEX_POINT('',#14241) ;
#3793=VERTEX_POINT('',#14243) ;
#3794=VERTEX_POINT('',#14248) ;
#4518=EDGE_CURVE('',#3641,#3642,#1019,.T.) ;
#4519=EDGE_CURVE('',#3642,#3641,#1020,.T.) ;
#4520=EDGE_CURVE('',#3643,#3644,#1021,.T.) ;
#4521=EDGE_CURVE('',#3644,#3645,#1022,.T.) ;
#4522=EDGE_CURVE('',#3645,#3643,#1023,.T.) ;
#4523=EDGE_CURVE('',#3646,#3647,#1024,.T.) ;
#4524=EDGE_CURVE('',#3647,#3648,#1025,.T.) ;
#4525=EDGE_CURVE('',#3648,#3649,#1026,.T.) ;
#4526=EDGE_CURVE('',#3649,#3646,#1027,.T.) ;
#4527=EDGE_CURVE('',#3650,#3651,#1028,.T.) ;
#4528=EDGE_CURVE('',#3651,#3652,#1029,.T.) ;
#4529=EDGE_CURVE('',#3652,#3653,#1030,.T.) ;
#4530=EDGE_CURVE('',#3653,#3650,#1031,.T.) ;
#4531=EDGE_CURVE('',#3654,#3655,#1032,.T.) ;
#4532=EDGE_CURVE('',#3655,#3656,#1033,.T.) ;
#4533=EDGE_CURVE('',#3656,#3657,#1034,.T.) ;
#4534=EDGE_CURVE('',#3657,#3654,#1035,.T.) ;
#4535=EDGE_CURVE('',#3658,#3659,#1036,.T.) ;
#4536=EDGE_CURVE('',#3659,#3660,#1037,.T.) ;
#4537=EDGE_CURVE('',#3660,#3658,#1038,.T.) ;
#4538=EDGE_CURVE('',#3661,#3662,#1039,.T.) ;
#4539=EDGE_CURVE('',#3662,#3661,#1040,.T.) ;
#4540=EDGE_CURVE('',#3663,#3664,#1041,.T.) ;
#4541=EDGE_CURVE('',#3664,#3663,#1042,.T.) ;
#4542=EDGE_CURVE('',#3665,#3666,#1043,.T.) ;
#4543=EDGE_CURVE('',#3666,#3665,#1044,.T.) ;
#4544=EDGE_CURVE('',#3667,#3668,#1045,.T.) ;
#4545=EDGE_CURVE('',#3668,#3669,#1046,.T.) ;
#4546=EDGE_CURVE('',#3669,#3667,#1047,.T.) ;
#4547=EDGE_CURVE('',#3670,#3671,#1048,.T.) ;
#4548=EDGE_CURVE('',#3671,#3672,#1049,.T.) ;
#4549=EDGE_CURVE('',#3672,#3673,#1050,.T.) ;
#4550=EDGE_CURVE('',#3673,#3670,#1051,.T.) ;
#4551=EDGE_CURVE('',#3674,#3675,#1052,.T.) ;
#4552=EDGE_CURVE('',#3675,#3676,#1053,.T.) ;
#4553=EDGE_CURVE('',#3676,#3677,#1054,.T.) ;
#4554=EDGE_CURVE('',#3677,#3674,#1055,.T.) ;
#4555=EDGE_CURVE('',#3678,#3679,#1056,.T.) ;
#4556=EDGE_CURVE('',#3679,#3680,#1057,.T.) ;
#4557=EDGE_CURVE('',#3680,#3681,#1058,.T.) ;
#4558=EDGE_CURVE('',#3681,#3678,#1059,.T.) ;
#4559=EDGE_CURVE('',#3682,#3683,#1060,.T.) ;
#4560=EDGE_CURVE('',#3683,#3684,#1061,.T.) ;
#4561=EDGE_CURVE('',#3684,#3682,#1062,.T.) ;
#4562=EDGE_CURVE('',#3685,#3686,#1063,.T.) ;
#4563=EDGE_CURVE('',#3686,#3685,#1064,.T.) ;
#4564=EDGE_CURVE('',#3687,#3688,#1065,.T.) ;
#4565=EDGE_CURVE('',#3688,#3687,#1066,.T.) ;
#4566=EDGE_CURVE('',#3689,#3690,#1067,.T.) ;
#4567=EDGE_CURVE('',#3690,#3689,#1068,.T.) ;
#4568=EDGE_CURVE('',#3691,#3692,#1069,.T.) ;
#4569=EDGE_CURVE('',#3692,#3693,#1070,.T.) ;
#4570=EDGE_CURVE('',#3693,#3691,#1071,.T.) ;
#4571=EDGE_CURVE('',#3694,#3695,#1072,.T.) ;
#4572=EDGE_CURVE('',#3695,#3696,#1073,.T.) ;
#4573=EDGE_CURVE('',#3696,#3697,#1074,.T.) ;
#4574=EDGE_CURVE('',#3697,#3694,#1075,.T.) ;
#4575=EDGE_CURVE('',#3698,#3699,#1076,.T.) ;
#4576=EDGE_CURVE('',#3699,#3700,#1077,.T.) ;
#4577=EDGE_CURVE('',#3700,#3701,#1078,.T.) ;
#4578=EDGE_CURVE('',#3701,#3698,#1079,.T.) ;
#4579=EDGE_CURVE('',#3702,#3703,#1080,.T.) ;
#4580=EDGE_CURVE('',#3703,#3704,#1081,.T.) ;
#4581=EDGE_CURVE('',#3704,#3705,#1082,.T.) ;
#4582=EDGE_CURVE('',#3705,#3702,#1083,.T.) ;
#4583=EDGE_CURVE('',#3706,#3707,#1084,.T.) ;
#4584=EDGE_CURVE('',#3707,#3708,#1085,.T.) ;
#4585=EDGE_CURVE('',#3708,#3706,#1086,.T.) ;
#4586=EDGE_CURVE('',#3709,#3710,#1087,.T.) ;
#4587=EDGE_CURVE('',#3710,#3709,#1088,.T.) ;
#4588=EDGE_CURVE('',#3711,#3712,#1089,.T.) ;
#4589=EDGE_CURVE('',#3712,#3711,#1090,.T.) ;
#4590=EDGE_CURVE('',#3713,#3714,#1091,.T.) ;
#4591=EDGE_CURVE('',#3714,#3713,#1092,.T.) ;
#4592=EDGE_CURVE('',#3715,#3716,#1093,.T.) ;
#4593=EDGE_CURVE('',#3716,#3717,#1094,.T.) ;
#4594=EDGE_CURVE('',#3717,#3715,#1095,.T.) ;
#4595=EDGE_CURVE('',#3718,#3719,#1096,.T.) ;
#4596=EDGE_CURVE('',#3719,#3720,#1097,.T.) ;
#4597=EDGE_CURVE('',#3720,#3721,#1098,.T.) ;
#4598=EDGE_CURVE('',#3721,#3718,#1099,.T.) ;
#4599=EDGE_CURVE('',#3722,#3723,#1100,.T.) ;
#4600=EDGE_CURVE('',#3723,#3724,#1101,.T.) ;
#4601=EDGE_CURVE('',#3724,#3725,#1102,.T.) ;
#4602=EDGE_CURVE('',#3725,#3722,#1103,.T.) ;
#4603=EDGE_CURVE('',#3726,#3727,#1104,.T.) ;
#4604=EDGE_CURVE('',#3727,#3728,#1105,.T.) ;
#4605=EDGE_CURVE('',#3728,#3729,#1106,.T.) ;
#4606=EDGE_CURVE('',#3729,#3726,#1107,.T.) ;
#4607=EDGE_CURVE('',#3730,#3731,#1108,.T.) ;
#4608=EDGE_CURVE('',#3731,#3732,#1109,.T.) ;
#4609=EDGE_CURVE('',#3732,#3730,#1110,.T.) ;
#4610=EDGE_CURVE('',#3733,#3734,#1111,.T.) ;
#4611=EDGE_CURVE('',#3734,#3733,#1112,.T.) ;
#4612=EDGE_CURVE('',#3735,#3736,#1113,.T.) ;
#4613=EDGE_CURVE('',#3736,#3735,#1114,.T.) ;
#4614=EDGE_CURVE('',#3737,#3738,#1115,.T.) ;
#4615=EDGE_CURVE('',#3738,#3737,#1116,.T.) ;
#4616=EDGE_CURVE('',#3739,#3740,#1117,.T.) ;
#4617=EDGE_CURVE('',#3740,#3741,#1118,.T.) ;
#4618=EDGE_CURVE('',#3741,#3739,#1119,.T.) ;
#4619=EDGE_CURVE('',#3742,#3743,#1120,.T.) ;
#4620=EDGE_CURVE('',#3743,#3744,#1121,.T.) ;
#4621=EDGE_CURVE('',#3744,#3745,#1122,.T.) ;
#4622=EDGE_CURVE('',#3745,#3742,#1123,.T.) ;
#4623=EDGE_CURVE('',#3746,#3747,#1124,.T.) ;
#4624=EDGE_CURVE('',#3747,#3748,#1125,.T.) ;
#4625=EDGE_CURVE('',#3748,#3749,#1126,.T.) ;
#4626=EDGE_CURVE('',#3749,#3746,#1127,.T.) ;
#4627=EDGE_CURVE('',#3750,#3751,#1128,.T.) ;
#4628=EDGE_CURVE('',#3751,#3752,#1129,.T.) ;
#4629=EDGE_CURVE('',#3752,#3753,#1130,.T.) ;
#4630=EDGE_CURVE('',#3753,#3750,#1131,.T.) ;
#4631=EDGE_CURVE('',#3754,#3755,#1132,.T.) ;
#4632=EDGE_CURVE('',#3755,#3756,#1133,.T.) ;
#4633=EDGE_CURVE('',#3756,#3754,#1134,.T.) ;
#4634=EDGE_CURVE('',#3757,#3758,#1135,.T.) ;
#4635=EDGE_CURVE('',#3758,#3757,#1136,.T.) ;
#4636=EDGE_CURVE('',#3759,#3759,#1137,.T.) ;
#4637=EDGE_CURVE('',#3759,#3760,#2679,.T.) ;
#4638=EDGE_CURVE('',#3761,#3760,#15,.T.) ;
#4639=EDGE_CURVE('',#3642,#3761,#16,.T.) ;
#4640=EDGE_CURVE('',#3760,#3641,#17,.T.) ;
#4641=EDGE_CURVE('',#3761,#3762,#2680,.T.) ;
#4642=EDGE_CURVE('',#3644,#3762,#18,.T.) ;
#4643=EDGE_CURVE('',#3762,#3643,#19,.T.) ;
#4644=EDGE_CURVE('',#3645,#3647,#2681,.T.) ;
#4645=EDGE_CURVE('',#3648,#3646,#20,.T.) ;
#4646=EDGE_CURVE('',#3649,#3651,#2682,.T.) ;
#4647=EDGE_CURVE('',#3652,#3650,#21,.T.) ;
#4648=EDGE_CURVE('',#3653,#3655,#2683,.T.) ;
#4649=EDGE_CURVE('',#3656,#3654,#22,.T.) ;
#4650=EDGE_CURVE('',#3657,#3659,#2684,.T.) ;
#4651=EDGE_CURVE('',#3763,#3658,#23,.T.) ;
#4652=EDGE_CURVE('',#3660,#3763,#24,.T.) ;
#4653=EDGE_CURVE('',#3763,#3764,#2685,.T.) ;
#4654=EDGE_CURVE('',#3765,#3764,#25,.T.) ;
#4655=EDGE_CURVE('',#3662,#3765,#26,.T.) ;
#4656=EDGE_CURVE('',#3764,#3661,#27,.T.) ;
#4657=EDGE_CURVE('',#3765,#3766,#2686,.T.) ;
#4658=EDGE_CURVE('',#3664,#3766,#28,.T.) ;
#4659=EDGE_CURVE('',#3766,#3663,#29,.T.) ;
#4660=EDGE_CURVE('',#3766,#3767,#2687,.T.) ;
#4661=EDGE_CURVE('',#3768,#3767,#30,.T.) ;
#4662=EDGE_CURVE('',#3666,#3768,#31,.T.) ;
#4663=EDGE_CURVE('',#3767,#3665,#32,.T.) ;
#4664=EDGE_CURVE('',#3768,#3769,#2688,.T.) ;
#4665=EDGE_CURVE('',#3668,#3769,#33,.T.) ;
#4666=EDGE_CURVE('',#3769,#3667,#34,.T.) ;
#4667=EDGE_CURVE('',#3669,#3671,#2689,.T.) ;
#4668=EDGE_CURVE('',#3672,#3670,#35,.T.) ;
#4669=EDGE_CURVE('',#3673,#3675,#2690,.T.) ;
#4670=EDGE_CURVE('',#3676,#3674,#36,.T.) ;
#4671=EDGE_CURVE('',#3677,#3679,#2691,.T.) ;
#4672=EDGE_CURVE('',#3680,#3678,#37,.T.) ;
#4673=EDGE_CURVE('',#3681,#3683,#2692,.T.) ;
#4674=EDGE_CURVE('',#3770,#3682,#38,.T.) ;
#4675=EDGE_CURVE('',#3684,#3770,#39,.T.) ;
#4676=EDGE_CURVE('',#3770,#3771,#2693,.T.) ;
#4677=EDGE_CURVE('',#3772,#3771,#40,.T.) ;
#4678=EDGE_CURVE('',#3686,#3772,#41,.T.) ;
#4679=EDGE_CURVE('',#3771,#3685,#42,.T.) ;
#4680=EDGE_CURVE('',#3772,#3773,#2694,.T.) ;
#4681=EDGE_CURVE('',#3688,#3773,#43,.T.) ;
#4682=EDGE_CURVE('',#3773,#3687,#44,.T.) ;
#4683=EDGE_CURVE('',#3773,#3774,#2695,.T.) ;
#4684=EDGE_CURVE('',#3775,#3774,#45,.T.) ;
#4685=EDGE_CURVE('',#3690,#3775,#46,.T.) ;
#4686=EDGE_CURVE('',#3774,#3689,#47,.T.) ;
#4687=EDGE_CURVE('',#3775,#3776,#2696,.T.) ;
#4688=EDGE_CURVE('',#3692,#3776,#48,.T.) ;
#4689=EDGE_CURVE('',#3776,#3691,#49,.T.) ;
#4690=EDGE_CURVE('',#3693,#3695,#2697,.T.) ;
#4691=EDGE_CURVE('',#3696,#3694,#50,.T.) ;
#4692=EDGE_CURVE('',#3697,#3699,#2698,.T.) ;
#4693=EDGE_CURVE('',#3700,#3698,#51,.T.) ;
#4694=EDGE_CURVE('',#3701,#3703,#2699,.T.) ;
#4695=EDGE_CURVE('',#3704,#3702,#52,.T.) ;
#4696=EDGE_CURVE('',#3705,#3707,#2700,.T.) ;
#4697=EDGE_CURVE('',#3777,#3706,#53,.T.) ;
#4698=EDGE_CURVE('',#3708,#3777,#54,.T.) ;
#4699=EDGE_CURVE('',#3777,#3778,#2701,.T.) ;
#4700=EDGE_CURVE('',#3779,#3778,#55,.T.) ;
#4701=EDGE_CURVE('',#3710,#3779,#56,.T.) ;
#4702=EDGE_CURVE('',#3778,#3709,#57,.T.) ;
#4703=EDGE_CURVE('',#3779,#3780,#2702,.T.) ;
#4704=EDGE_CURVE('',#3712,#3780,#58,.T.) ;
#4705=EDGE_CURVE('',#3780,#3711,#59,.T.) ;
#4706=EDGE_CURVE('',#3780,#3781,#2703,.T.) ;
#4707=EDGE_CURVE('',#3782,#3781,#60,.T.) ;
#4708=EDGE_CURVE('',#3714,#3782,#61,.T.) ;
#4709=EDGE_CURVE('',#3781,#3713,#62,.T.) ;
#4710=EDGE_CURVE('',#3782,#3783,#2704,.T.) ;
#4711=EDGE_CURVE('',#3716,#3783,#63,.T.) ;
#4712=EDGE_CURVE('',#3783,#3715,#64,.T.) ;
#4713=EDGE_CURVE('',#3717,#3719,#2705,.T.) ;
#4714=EDGE_CURVE('',#3720,#3718,#65,.T.) ;
#4715=EDGE_CURVE('',#3721,#3723,#2706,.T.) ;
#4716=EDGE_CURVE('',#3724,#3722,#66,.T.) ;
#4717=EDGE_CURVE('',#3725,#3727,#2707,.T.) ;
#4718=EDGE_CURVE('',#3728,#3726,#67,.T.) ;
#4719=EDGE_CURVE('',#3729,#3731,#2708,.T.) ;
#4720=EDGE_CURVE('',#3784,#3730,#68,.T.) ;
#4721=EDGE_CURVE('',#3732,#3784,#69,.T.) ;
#4722=EDGE_CURVE('',#3784,#3785,#2709,.T.) ;
#4723=EDGE_CURVE('',#3786,#3785,#70,.T.) ;
#4724=EDGE_CURVE('',#3734,#3786,#71,.T.) ;
#4725=EDGE_CURVE('',#3785,#3733,#72,.T.) ;
#4726=EDGE_CURVE('',#3786,#3787,#2710,.T.) ;
#4727=EDGE_CURVE('',#3736,#3787,#73,.T.) ;
#4728=EDGE_CURVE('',#3787,#3735,#74,.T.) ;
#4729=EDGE_CURVE('',#3787,#3788,#2711,.T.) ;
#4730=EDGE_CURVE('',#3789,#3788,#75,.T.) ;
#4731=EDGE_CURVE('',#3738,#3789,#76,.T.) ;
#4732=EDGE_CURVE('',#3788,#3737,#77,.T.) ;
#4733=EDGE_CURVE('',#3789,#3790,#2712,.T.) ;
#4734=EDGE_CURVE('',#3740,#3790,#78,.T.) ;
#4735=EDGE_CURVE('',#3790,#3739,#79,.T.) ;
#4736=EDGE_CURVE('',#3741,#3743,#2713,.T.) ;
#4737=EDGE_CURVE('',#3744,#3742,#80,.T.) ;
#4738=EDGE_CURVE('',#3745,#3747,#2714,.T.) ;
#4739=EDGE_CURVE('',#3748,#3746,#81,.T.) ;
#4740=EDGE_CURVE('',#3749,#3751,#2715,.T.) ;
#4741=EDGE_CURVE('',#3752,#3750,#82,.T.) ;
#4742=EDGE_CURVE('',#3753,#3755,#2716,.T.) ;
#4743=EDGE_CURVE('',#3791,#3754,#83,.T.) ;
#4744=EDGE_CURVE('',#3756,#3791,#84,.T.) ;
#4745=EDGE_CURVE('',#3791,#3792,#2717,.T.) ;
#4746=EDGE_CURVE('',#3793,#3792,#85,.T.) ;
#4747=EDGE_CURVE('',#3758,#3793,#86,.T.) ;
#4748=EDGE_CURVE('',#3792,#3757,#87,.T.) ;
#4749=EDGE_CURVE('',#3793,#3794,#2718,.T.) ;
#4750=EDGE_CURVE('',#3794,#3794,#1138,.T.) ;
#6027=ORIENTED_EDGE('',*,*,#4518,.T.) ;
#6028=ORIENTED_EDGE('',*,*,#4519,.T.) ;
#6029=ORIENTED_EDGE('',*,*,#4520,.T.) ;
#6030=ORIENTED_EDGE('',*,*,#4521,.T.) ;
#6031=ORIENTED_EDGE('',*,*,#4522,.T.) ;
#6032=ORIENTED_EDGE('',*,*,#4523,.T.) ;
#6033=ORIENTED_EDGE('',*,*,#4524,.T.) ;
#6034=ORIENTED_EDGE('',*,*,#4525,.T.) ;
#6035=ORIENTED_EDGE('',*,*,#4526,.T.) ;
#6036=ORIENTED_EDGE('',*,*,#4527,.T.) ;
#6037=ORIENTED_EDGE('',*,*,#4528,.T.) ;
#6038=ORIENTED_EDGE('',*,*,#4529,.T.) ;
#6039=ORIENTED_EDGE('',*,*,#4530,.T.) ;
#6040=ORIENTED_EDGE('',*,*,#4531,.T.) ;
#6041=ORIENTED_EDGE('',*,*,#4532,.T.) ;
#6042=ORIENTED_EDGE('',*,*,#4533,.T.) ;
#6043=ORIENTED_EDGE('',*,*,#4534,.T.) ;
#6044=ORIENTED_EDGE('',*,*,#4535,.T.) ;
#6045=ORIENTED_EDGE('',*,*,#4536,.T.) ;
#6046=ORIENTED_EDGE('',*,*,#4537,.T.) ;
#6047=ORIENTED_EDGE('',*,*,#4538,.T.) ;
#6048=ORIENTED_EDGE('',*,*,#4539,.T.) ;
#6049=ORIENTED_EDGE('',*,*,#4540,.T.) ;
#6050=ORIENTED_EDGE('',*,*,#4541,.T.) ;
#6051=ORIENTED_EDGE('',*,*,#4542,.T.) ;
#6052=ORIENTED_EDGE('',*,*,#4543,.T.) ;
#6053=ORIENTED_EDGE('',*,*,#4544,.T.) ;
#6054=ORIENTED_EDGE('',*,*,#4545,.T.) ;
#6055=ORIENTED_EDGE('',*,*,#4546,.T.) ;
#6056=ORIENTED_EDGE('',*,*,#4547,.T.) ;
#6057=ORIENTED_EDGE('',*,*,#4548,.T.) ;
#6058=ORIENTED_EDGE('',*,*,#4549,.T.) ;
#6059=ORIENTED_EDGE('',*,*,#4550,.T.) ;
#6060=ORIENTED_EDGE('',*,*,#4551,.T.) ;
#6061=ORIENTED_EDGE('',*,*,#4552,.T.) ;
#6062=ORIENTED_EDGE('',*,*,#4553,.T.) ;
#6063=ORIENTED_EDGE('',*,*,#4554,.T.) ;
#6064=ORIENTED_EDGE('',*,*,#4555,.T.) ;
#6065=ORIENTED_EDGE('',*,*,#4556,.T.) ;
#6066=ORIENTED_EDGE('',*,*,#4557,.T.) ;
#6067=ORIENTED_EDGE('',*,*,#4558,.T.) ;
#6068=ORIENTED_EDGE('',*,*,#4559,.T.) ;
#6069=ORIENTED_EDGE('',*,*,#4560,.T.) ;
#6070=ORIENTED_EDGE('',*,*,#4561,.T.) ;
#6071=ORIENTED_EDGE('',*,*,#4562,.T.) ;
#6072=ORIENTED_EDGE('',*,*,#4563,.T.) ;
#6073=ORIENTED_EDGE('',*,*,#4564,.T.) ;
#6074=ORIENTED_EDGE('',*,*,#4565,.T.) ;
#6075=ORIENTED_EDGE('',*,*,#4566,.T.) ;
#6076=ORIENTED_EDGE('',*,*,#4567,.T.) ;
#6077=ORIENTED_EDGE('',*,*,#4568,.T.) ;
#6078=ORIENTED_EDGE('',*,*,#4569,.T.) ;
#6079=ORIENTED_EDGE('',*,*,#4570,.T.) ;
#6080=ORIENTED_EDGE('',*,*,#4571,.T.) ;
#6081=ORIENTED_EDGE('',*,*,#4572,.T.) ;
#6082=ORIENTED_EDGE('',*,*,#4573,.T.) ;
#6083=ORIENTED_EDGE('',*,*,#4574,.T.) ;
#6084=ORIENTED_EDGE('',*,*,#4575,.T.) ;
#6085=ORIENTED_EDGE('',*,*,#4576,.T.) ;
#6086=ORIENTED_EDGE('',*,*,#4577,.T.) ;
#6087=ORIENTED_EDGE('',*,*,#4578,.T.) ;
#6088=ORIENTED_EDGE('',*,*,#4579,.T.) ;
#6089=ORIENTED_EDGE('',*,*,#4580,.T.) ;
#6090=ORIENTED_EDGE('',*,*,#4581,.T.) ;
#6091=ORIENTED_EDGE('',*,*,#4582,.T.) ;
#6092=ORIENTED_EDGE('',*,*,#4583,.T.) ;
#6093=ORIENTED_EDGE('',*,*,#4584,.T.) ;
#6094=ORIENTED_EDGE('',*,*,#4585,.T.) ;
#6095=ORIENTED_EDGE('',*,*,#4586,.T.) ;
#6096=ORIENTED_EDGE('',*,*,#4587,.T.) ;
#6097=ORIENTED_EDGE('',*,*,#4588,.T.) ;
#6098=ORIENTED_EDGE('',*,*,#4589,.T.) ;
#6099=ORIENTED_EDGE('',*,*,#4590,.T.) ;
#6100=ORIENTED_EDGE('',*,*,#4591,.T.) ;
#6101=ORIENTED_EDGE('',*,*,#4592,.T.) ;
#6102=ORIENTED_EDGE('',*,*,#4593,.T.) ;
#6103=ORIENTED_EDGE('',*,*,#4594,.T.) ;
#6104=ORIENTED_EDGE('',*,*,#4595,.T.) ;
#6105=ORIENTED_EDGE('',*,*,#4596,.T.) ;
#6106=ORIENTED_EDGE('',*,*,#4597,.T.) ;
#6107=ORIENTED_EDGE('',*,*,#4598,.T.) ;
#6108=ORIENTED_EDGE('',*,*,#4599,.T.) ;
#6109=ORIENTED_EDGE('',*,*,#4600,.T.) ;
#6110=ORIENTED_EDGE('',*,*,#4601,.T.) ;
#6111=ORIENTED_EDGE('',*,*,#4602,.T.) ;
#6112=ORIENTED_EDGE('',*,*,#4603,.T.) ;
#6113=ORIENTED_EDGE('',*,*,#4604,.T.) ;
#6114=ORIENTED_EDGE('',*,*,#4605,.T.) ;
#6115=ORIENTED_EDGE('',*,*,#4606,.T.) ;
#6116=ORIENTED_EDGE('',*,*,#4607,.T.) ;
#6117=ORIENTED_EDGE('',*,*,#4608,.T.) ;
#6118=ORIENTED_EDGE('',*,*,#4609,.T.) ;
#6119=ORIENTED_EDGE('',*,*,#4610,.T.) ;
#6120=ORIENTED_EDGE('',*,*,#4611,.T.) ;
#6121=ORIENTED_EDGE('',*,*,#4612,.T.) ;
#6122=ORIENTED_EDGE('',*,*,#4613,.T.) ;
#6123=ORIENTED_EDGE('',*,*,#4614,.T.) ;
#6124=ORIENTED_EDGE('',*,*,#4615,.T.) ;
#6125=ORIENTED_EDGE('',*,*,#4616,.T.) ;
#6126=ORIENTED_EDGE('',*,*,#4617,.T.) ;
#6127=ORIENTED_EDGE('',*,*,#4618,.T.) ;
#6128=ORIENTED_EDGE('',*,*,#4619,.T.) ;
#6129=ORIENTED_EDGE('',*,*,#4620,.T.) ;
#6130=ORIENTED_EDGE('',*,*,#4621,.T.) ;
#6131=ORIENTED_EDGE('',*,*,#4622,.T.) ;
#6132=ORIENTED_EDGE('',*,*,#4623,.T.) ;
#6133=ORIENTED_EDGE('',*,*,#4624,.T.) ;
#6134=ORIENTED_EDGE('',*,*,#4625,.T.) ;
#6135=ORIENTED_EDGE('',*,*,#4626,.T.) ;
#6136=ORIENTED_EDGE('',*,*,#4627,.T.) ;
#6137=ORIENTED_EDGE('',*,*,#4628,.T.) ;
#6138=ORIENTED_EDGE('',*,*,#4629,.T.) ;
#6139=ORIENTED_EDGE('',*,*,#4630,.T.) ;
#6140=ORIENTED_EDGE('',*,*,#4631,.T.) ;
#6141=ORIENTED_EDGE('',*,*,#4632,.T.) ;
#6142=ORIENTED_EDGE('',*,*,#4633,.T.) ;
#6143=ORIENTED_EDGE('',*,*,#4634,.T.) ;
#6144=ORIENTED_EDGE('',*,*,#4635,.T.) ;
#6145=ORIENTED_EDGE('',*,*,#4636,.F.) ;
#6146=ORIENTED_EDGE('',*,*,#4637,.T.) ;
#6147=ORIENTED_EDGE('',*,*,#4638,.F.) ;
#6148=ORIENTED_EDGE('',*,*,#4639,.F.) ;
#6149=ORIENTED_EDGE('',*,*,#4518,.F.) ;
#6150=ORIENTED_EDGE('',*,*,#4640,.F.) ;
#6151=ORIENTED_EDGE('',*,*,#4637,.F.) ;
#6152=ORIENTED_EDGE('',*,*,#4636,.T.) ;
#6153=ORIENTED_EDGE('',*,*,#4639,.T.) ;
#6154=ORIENTED_EDGE('',*,*,#4641,.T.) ;
#6155=ORIENTED_EDGE('',*,*,#4642,.F.) ;
#6156=ORIENTED_EDGE('',*,*,#4520,.F.) ;
#6157=ORIENTED_EDGE('',*,*,#4643,.F.) ;
#6158=ORIENTED_EDGE('',*,*,#4641,.F.) ;
#6159=ORIENTED_EDGE('',*,*,#4638,.T.) ;
#6160=ORIENTED_EDGE('',*,*,#4640,.T.) ;
#6161=ORIENTED_EDGE('',*,*,#4519,.F.) ;
#6162=ORIENTED_EDGE('',*,*,#4642,.T.) ;
#6163=ORIENTED_EDGE('',*,*,#4643,.T.) ;
#6164=ORIENTED_EDGE('',*,*,#4522,.F.) ;
#6165=ORIENTED_EDGE('',*,*,#4644,.T.) ;
#6166=ORIENTED_EDGE('',*,*,#4523,.F.) ;
#6167=ORIENTED_EDGE('',*,*,#4645,.F.) ;
#6168=ORIENTED_EDGE('',*,*,#4524,.F.) ;
#6169=ORIENTED_EDGE('',*,*,#4644,.F.) ;
#6170=ORIENTED_EDGE('',*,*,#4521,.F.) ;
#6171=ORIENTED_EDGE('',*,*,#4645,.T.) ;
#6172=ORIENTED_EDGE('',*,*,#4526,.F.) ;
#6173=ORIENTED_EDGE('',*,*,#4646,.T.) ;
#6174=ORIENTED_EDGE('',*,*,#4527,.F.) ;
#6175=ORIENTED_EDGE('',*,*,#4647,.F.) ;
#6176=ORIENTED_EDGE('',*,*,#4528,.F.) ;
#6177=ORIENTED_EDGE('',*,*,#4646,.F.) ;
#6178=ORIENTED_EDGE('',*,*,#4525,.F.) ;
#6179=ORIENTED_EDGE('',*,*,#4647,.T.) ;
#6180=ORIENTED_EDGE('',*,*,#4530,.F.) ;
#6181=ORIENTED_EDGE('',*,*,#4648,.T.) ;
#6182=ORIENTED_EDGE('',*,*,#4531,.F.) ;
#6183=ORIENTED_EDGE('',*,*,#4649,.F.) ;
#6184=ORIENTED_EDGE('',*,*,#4532,.F.) ;
#6185=ORIENTED_EDGE('',*,*,#4648,.F.) ;
#6186=ORIENTED_EDGE('',*,*,#4529,.F.) ;
#6187=ORIENTED_EDGE('',*,*,#4649,.T.) ;
#6188=ORIENTED_EDGE('',*,*,#4534,.F.) ;
#6189=ORIENTED_EDGE('',*,*,#4650,.T.) ;
#6190=ORIENTED_EDGE('',*,*,#4535,.F.) ;
#6191=ORIENTED_EDGE('',*,*,#4651,.F.) ;
#6192=ORIENTED_EDGE('',*,*,#4652,.F.) ;
#6193=ORIENTED_EDGE('',*,*,#4536,.F.) ;
#6194=ORIENTED_EDGE('',*,*,#4650,.F.) ;
#6195=ORIENTED_EDGE('',*,*,#4533,.F.) ;
#6196=ORIENTED_EDGE('',*,*,#4652,.T.) ;
#6197=ORIENTED_EDGE('',*,*,#4653,.T.) ;
#6198=ORIENTED_EDGE('',*,*,#4654,.F.) ;
#6199=ORIENTED_EDGE('',*,*,#4655,.F.) ;
#6200=ORIENTED_EDGE('',*,*,#4538,.F.) ;
#6201=ORIENTED_EDGE('',*,*,#4656,.F.) ;
#6202=ORIENTED_EDGE('',*,*,#4653,.F.) ;
#6203=ORIENTED_EDGE('',*,*,#4651,.T.) ;
#6204=ORIENTED_EDGE('',*,*,#4537,.F.) ;
#6205=ORIENTED_EDGE('',*,*,#4655,.T.) ;
#6206=ORIENTED_EDGE('',*,*,#4657,.T.) ;
#6207=ORIENTED_EDGE('',*,*,#4658,.F.) ;
#6208=ORIENTED_EDGE('',*,*,#4540,.F.) ;
#6209=ORIENTED_EDGE('',*,*,#4659,.F.) ;
#6210=ORIENTED_EDGE('',*,*,#4657,.F.) ;
#6211=ORIENTED_EDGE('',*,*,#4654,.T.) ;
#6212=ORIENTED_EDGE('',*,*,#4656,.T.) ;
#6213=ORIENTED_EDGE('',*,*,#4539,.F.) ;
#6214=ORIENTED_EDGE('',*,*,#4658,.T.) ;
#6215=ORIENTED_EDGE('',*,*,#4660,.T.) ;
#6216=ORIENTED_EDGE('',*,*,#4661,.F.) ;
#6217=ORIENTED_EDGE('',*,*,#4662,.F.) ;
#6218=ORIENTED_EDGE('',*,*,#4542,.F.) ;
#6219=ORIENTED_EDGE('',*,*,#4663,.F.) ;
#6220=ORIENTED_EDGE('',*,*,#4660,.F.) ;
#6221=ORIENTED_EDGE('',*,*,#4659,.T.) ;
#6222=ORIENTED_EDGE('',*,*,#4541,.F.) ;
#6223=ORIENTED_EDGE('',*,*,#4662,.T.) ;
#6224=ORIENTED_EDGE('',*,*,#4664,.T.) ;
#6225=ORIENTED_EDGE('',*,*,#4665,.F.) ;
#6226=ORIENTED_EDGE('',*,*,#4544,.F.) ;
#6227=ORIENTED_EDGE('',*,*,#4666,.F.) ;
#6228=ORIENTED_EDGE('',*,*,#4664,.F.) ;
#6229=ORIENTED_EDGE('',*,*,#4661,.T.) ;
#6230=ORIENTED_EDGE('',*,*,#4663,.T.) ;
#6231=ORIENTED_EDGE('',*,*,#4543,.F.) ;
#6232=ORIENTED_EDGE('',*,*,#4665,.T.) ;
#6233=ORIENTED_EDGE('',*,*,#4666,.T.) ;
#6234=ORIENTED_EDGE('',*,*,#4546,.F.) ;
#6235=ORIENTED_EDGE('',*,*,#4667,.T.) ;
#6236=ORIENTED_EDGE('',*,*,#4547,.F.) ;
#6237=ORIENTED_EDGE('',*,*,#4668,.F.) ;
#6238=ORIENTED_EDGE('',*,*,#4548,.F.) ;
#6239=ORIENTED_EDGE('',*,*,#4667,.F.) ;
#6240=ORIENTED_EDGE('',*,*,#4545,.F.) ;
#6241=ORIENTED_EDGE('',*,*,#4668,.T.) ;
#6242=ORIENTED_EDGE('',*,*,#4550,.F.) ;
#6243=ORIENTED_EDGE('',*,*,#4669,.T.) ;
#6244=ORIENTED_EDGE('',*,*,#4551,.F.) ;
#6245=ORIENTED_EDGE('',*,*,#4670,.F.) ;
#6246=ORIENTED_EDGE('',*,*,#4552,.F.) ;
#6247=ORIENTED_EDGE('',*,*,#4669,.F.) ;
#6248=ORIENTED_EDGE('',*,*,#4549,.F.) ;
#6249=ORIENTED_EDGE('',*,*,#4670,.T.) ;
#6250=ORIENTED_EDGE('',*,*,#4554,.F.) ;
#6251=ORIENTED_EDGE('',*,*,#4671,.T.) ;
#6252=ORIENTED_EDGE('',*,*,#4555,.F.) ;
#6253=ORIENTED_EDGE('',*,*,#4672,.F.) ;
#6254=ORIENTED_EDGE('',*,*,#4556,.F.) ;
#6255=ORIENTED_EDGE('',*,*,#4671,.F.) ;
#6256=ORIENTED_EDGE('',*,*,#4553,.F.) ;
#6257=ORIENTED_EDGE('',*,*,#4672,.T.) ;
#6258=ORIENTED_EDGE('',*,*,#4558,.F.) ;
#6259=ORIENTED_EDGE('',*,*,#4673,.T.) ;
#6260=ORIENTED_EDGE('',*,*,#4559,.F.) ;
#6261=ORIENTED_EDGE('',*,*,#4674,.F.) ;
#6262=ORIENTED_EDGE('',*,*,#4675,.F.) ;
#6263=ORIENTED_EDGE('',*,*,#4560,.F.) ;
#6264=ORIENTED_EDGE('',*,*,#4673,.F.) ;
#6265=ORIENTED_EDGE('',*,*,#4557,.F.) ;
#6266=ORIENTED_EDGE('',*,*,#4675,.T.) ;
#6267=ORIENTED_EDGE('',*,*,#4676,.T.) ;
#6268=ORIENTED_EDGE('',*,*,#4677,.F.) ;
#6269=ORIENTED_EDGE('',*,*,#4678,.F.) ;
#6270=ORIENTED_EDGE('',*,*,#4562,.F.) ;
#6271=ORIENTED_EDGE('',*,*,#4679,.F.) ;
#6272=ORIENTED_EDGE('',*,*,#4676,.F.) ;
#6273=ORIENTED_EDGE('',*,*,#4674,.T.) ;
#6274=ORIENTED_EDGE('',*,*,#4561,.F.) ;
#6275=ORIENTED_EDGE('',*,*,#4678,.T.) ;
#6276=ORIENTED_EDGE('',*,*,#4680,.T.) ;
#6277=ORIENTED_EDGE('',*,*,#4681,.F.) ;
#6278=ORIENTED_EDGE('',*,*,#4564,.F.) ;
#6279=ORIENTED_EDGE('',*,*,#4682,.F.) ;
#6280=ORIENTED_EDGE('',*,*,#4680,.F.) ;
#6281=ORIENTED_EDGE('',*,*,#4677,.T.) ;
#6282=ORIENTED_EDGE('',*,*,#4679,.T.) ;
#6283=ORIENTED_EDGE('',*,*,#4563,.F.) ;
#6284=ORIENTED_EDGE('',*,*,#4681,.T.) ;
#6285=ORIENTED_EDGE('',*,*,#4683,.T.) ;
#6286=ORIENTED_EDGE('',*,*,#4684,.F.) ;
#6287=ORIENTED_EDGE('',*,*,#4685,.F.) ;
#6288=ORIENTED_EDGE('',*,*,#4566,.F.) ;
#6289=ORIENTED_EDGE('',*,*,#4686,.F.) ;
#6290=ORIENTED_EDGE('',*,*,#4683,.F.) ;
#6291=ORIENTED_EDGE('',*,*,#4682,.T.) ;
#6292=ORIENTED_EDGE('',*,*,#4565,.F.) ;
#6293=ORIENTED_EDGE('',*,*,#4685,.T.) ;
#6294=ORIENTED_EDGE('',*,*,#4687,.T.) ;
#6295=ORIENTED_EDGE('',*,*,#4688,.F.) ;
#6296=ORIENTED_EDGE('',*,*,#4568,.F.) ;
#6297=ORIENTED_EDGE('',*,*,#4689,.F.) ;
#6298=ORIENTED_EDGE('',*,*,#4687,.F.) ;
#6299=ORIENTED_EDGE('',*,*,#4684,.T.) ;
#6300=ORIENTED_EDGE('',*,*,#4686,.T.) ;
#6301=ORIENTED_EDGE('',*,*,#4567,.F.) ;
#6302=ORIENTED_EDGE('',*,*,#4688,.T.) ;
#6303=ORIENTED_EDGE('',*,*,#4689,.T.) ;
#6304=ORIENTED_EDGE('',*,*,#4570,.F.) ;
#6305=ORIENTED_EDGE('',*,*,#4690,.T.) ;
#6306=ORIENTED_EDGE('',*,*,#4571,.F.) ;
#6307=ORIENTED_EDGE('',*,*,#4691,.F.) ;
#6308=ORIENTED_EDGE('',*,*,#4572,.F.) ;
#6309=ORIENTED_EDGE('',*,*,#4690,.F.) ;
#6310=ORIENTED_EDGE('',*,*,#4569,.F.) ;
#6311=ORIENTED_EDGE('',*,*,#4691,.T.) ;
#6312=ORIENTED_EDGE('',*,*,#4574,.F.) ;
#6313=ORIENTED_EDGE('',*,*,#4692,.T.) ;
#6314=ORIENTED_EDGE('',*,*,#4575,.F.) ;
#6315=ORIENTED_EDGE('',*,*,#4693,.F.) ;
#6316=ORIENTED_EDGE('',*,*,#4576,.F.) ;
#6317=ORIENTED_EDGE('',*,*,#4692,.F.) ;
#6318=ORIENTED_EDGE('',*,*,#4573,.F.) ;
#6319=ORIENTED_EDGE('',*,*,#4693,.T.) ;
#6320=ORIENTED_EDGE('',*,*,#4578,.F.) ;
#6321=ORIENTED_EDGE('',*,*,#4694,.T.) ;
#6322=ORIENTED_EDGE('',*,*,#4579,.F.) ;
#6323=ORIENTED_EDGE('',*,*,#4695,.F.) ;
#6324=ORIENTED_EDGE('',*,*,#4580,.F.) ;
#6325=ORIENTED_EDGE('',*,*,#4694,.F.) ;
#6326=ORIENTED_EDGE('',*,*,#4577,.F.) ;
#6327=ORIENTED_EDGE('',*,*,#4695,.T.) ;
#6328=ORIENTED_EDGE('',*,*,#4582,.F.) ;
#6329=ORIENTED_EDGE('',*,*,#4696,.T.) ;
#6330=ORIENTED_EDGE('',*,*,#4583,.F.) ;
#6331=ORIENTED_EDGE('',*,*,#4697,.F.) ;
#6332=ORIENTED_EDGE('',*,*,#4698,.F.) ;
#6333=ORIENTED_EDGE('',*,*,#4584,.F.) ;
#6334=ORIENTED_EDGE('',*,*,#4696,.F.) ;
#6335=ORIENTED_EDGE('',*,*,#4581,.F.) ;
#6336=ORIENTED_EDGE('',*,*,#4698,.T.) ;
#6337=ORIENTED_EDGE('',*,*,#4699,.T.) ;
#6338=ORIENTED_EDGE('',*,*,#4700,.F.) ;
#6339=ORIENTED_EDGE('',*,*,#4701,.F.) ;
#6340=ORIENTED_EDGE('',*,*,#4586,.F.) ;
#6341=ORIENTED_EDGE('',*,*,#4702,.F.) ;
#6342=ORIENTED_EDGE('',*,*,#4699,.F.) ;
#6343=ORIENTED_EDGE('',*,*,#4697,.T.) ;
#6344=ORIENTED_EDGE('',*,*,#4585,.F.) ;
#6345=ORIENTED_EDGE('',*,*,#4701,.T.) ;
#6346=ORIENTED_EDGE('',*,*,#4703,.T.) ;
#6347=ORIENTED_EDGE('',*,*,#4704,.F.) ;
#6348=ORIENTED_EDGE('',*,*,#4588,.F.) ;
#6349=ORIENTED_EDGE('',*,*,#4705,.F.) ;
#6350=ORIENTED_EDGE('',*,*,#4703,.F.) ;
#6351=ORIENTED_EDGE('',*,*,#4700,.T.) ;
#6352=ORIENTED_EDGE('',*,*,#4702,.T.) ;
#6353=ORIENTED_EDGE('',*,*,#4587,.F.) ;
#6354=ORIENTED_EDGE('',*,*,#4704,.T.) ;
#6355=ORIENTED_EDGE('',*,*,#4706,.T.) ;
#6356=ORIENTED_EDGE('',*,*,#4707,.F.) ;
#6357=ORIENTED_EDGE('',*,*,#4708,.F.) ;
#6358=ORIENTED_EDGE('',*,*,#4590,.F.) ;
#6359=ORIENTED_EDGE('',*,*,#4709,.F.) ;
#6360=ORIENTED_EDGE('',*,*,#4706,.F.) ;
#6361=ORIENTED_EDGE('',*,*,#4705,.T.) ;
#6362=ORIENTED_EDGE('',*,*,#4589,.F.) ;
#6363=ORIENTED_EDGE('',*,*,#4708,.T.) ;
#6364=ORIENTED_EDGE('',*,*,#4710,.T.) ;
#6365=ORIENTED_EDGE('',*,*,#4711,.F.) ;
#6366=ORIENTED_EDGE('',*,*,#4592,.F.) ;
#6367=ORIENTED_EDGE('',*,*,#4712,.F.) ;
#6368=ORIENTED_EDGE('',*,*,#4710,.F.) ;
#6369=ORIENTED_EDGE('',*,*,#4707,.T.) ;
#6370=ORIENTED_EDGE('',*,*,#4709,.T.) ;
#6371=ORIENTED_EDGE('',*,*,#4591,.F.) ;
#6372=ORIENTED_EDGE('',*,*,#4711,.T.) ;
#6373=ORIENTED_EDGE('',*,*,#4712,.T.) ;
#6374=ORIENTED_EDGE('',*,*,#4594,.F.) ;
#6375=ORIENTED_EDGE('',*,*,#4713,.T.) ;
#6376=ORIENTED_EDGE('',*,*,#4595,.F.) ;
#6377=ORIENTED_EDGE('',*,*,#4714,.F.) ;
#6378=ORIENTED_EDGE('',*,*,#4596,.F.) ;
#6379=ORIENTED_EDGE('',*,*,#4713,.F.) ;
#6380=ORIENTED_EDGE('',*,*,#4593,.F.) ;
#6381=ORIENTED_EDGE('',*,*,#4714,.T.) ;
#6382=ORIENTED_EDGE('',*,*,#4598,.F.) ;
#6383=ORIENTED_EDGE('',*,*,#4715,.T.) ;
#6384=ORIENTED_EDGE('',*,*,#4599,.F.) ;
#6385=ORIENTED_EDGE('',*,*,#4716,.F.) ;
#6386=ORIENTED_EDGE('',*,*,#4600,.F.) ;
#6387=ORIENTED_EDGE('',*,*,#4715,.F.) ;
#6388=ORIENTED_EDGE('',*,*,#4597,.F.) ;
#6389=ORIENTED_EDGE('',*,*,#4716,.T.) ;
#6390=ORIENTED_EDGE('',*,*,#4602,.F.) ;
#6391=ORIENTED_EDGE('',*,*,#4717,.T.) ;
#6392=ORIENTED_EDGE('',*,*,#4603,.F.) ;
#6393=ORIENTED_EDGE('',*,*,#4718,.F.) ;
#6394=ORIENTED_EDGE('',*,*,#4604,.F.) ;
#6395=ORIENTED_EDGE('',*,*,#4717,.F.) ;
#6396=ORIENTED_EDGE('',*,*,#4601,.F.) ;
#6397=ORIENTED_EDGE('',*,*,#4718,.T.) ;
#6398=ORIENTED_EDGE('',*,*,#4606,.F.) ;
#6399=ORIENTED_EDGE('',*,*,#4719,.T.) ;
#6400=ORIENTED_EDGE('',*,*,#4607,.F.) ;
#6401=ORIENTED_EDGE('',*,*,#4720,.F.) ;
#6402=ORIENTED_EDGE('',*,*,#4721,.F.) ;
#6403=ORIENTED_EDGE('',*,*,#4608,.F.) ;
#6404=ORIENTED_EDGE('',*,*,#4719,.F.) ;
#6405=ORIENTED_EDGE('',*,*,#4605,.F.) ;
#6406=ORIENTED_EDGE('',*,*,#4721,.T.) ;
#6407=ORIENTED_EDGE('',*,*,#4722,.T.) ;
#6408=ORIENTED_EDGE('',*,*,#4723,.F.) ;
#6409=ORIENTED_EDGE('',*,*,#4724,.F.) ;
#6410=ORIENTED_EDGE('',*,*,#4610,.F.) ;
#6411=ORIENTED_EDGE('',*,*,#4725,.F.) ;
#6412=ORIENTED_EDGE('',*,*,#4722,.F.) ;
#6413=ORIENTED_EDGE('',*,*,#4720,.T.) ;
#6414=ORIENTED_EDGE('',*,*,#4609,.F.) ;
#6415=ORIENTED_EDGE('',*,*,#4724,.T.) ;
#6416=ORIENTED_EDGE('',*,*,#4726,.T.) ;
#6417=ORIENTED_EDGE('',*,*,#4727,.F.) ;
#6418=ORIENTED_EDGE('',*,*,#4612,.F.) ;
#6419=ORIENTED_EDGE('',*,*,#4728,.F.) ;
#6420=ORIENTED_EDGE('',*,*,#4726,.F.) ;
#6421=ORIENTED_EDGE('',*,*,#4723,.T.) ;
#6422=ORIENTED_EDGE('',*,*,#4725,.T.) ;
#6423=ORIENTED_EDGE('',*,*,#4611,.F.) ;
#6424=ORIENTED_EDGE('',*,*,#4727,.T.) ;
#6425=ORIENTED_EDGE('',*,*,#4729,.T.) ;
#6426=ORIENTED_EDGE('',*,*,#4730,.F.) ;
#6427=ORIENTED_EDGE('',*,*,#4731,.F.) ;
#6428=ORIENTED_EDGE('',*,*,#4614,.F.) ;
#6429=ORIENTED_EDGE('',*,*,#4732,.F.) ;
#6430=ORIENTED_EDGE('',*,*,#4729,.F.) ;
#6431=ORIENTED_EDGE('',*,*,#4728,.T.) ;
#6432=ORIENTED_EDGE('',*,*,#4613,.F.) ;
#6433=ORIENTED_EDGE('',*,*,#4731,.T.) ;
#6434=ORIENTED_EDGE('',*,*,#4733,.T.) ;
#6435=ORIENTED_EDGE('',*,*,#4734,.F.) ;
#6436=ORIENTED_EDGE('',*,*,#4616,.F.) ;
#6437=ORIENTED_EDGE('',*,*,#4735,.F.) ;
#6438=ORIENTED_EDGE('',*,*,#4733,.F.) ;
#6439=ORIENTED_EDGE('',*,*,#4730,.T.) ;
#6440=ORIENTED_EDGE('',*,*,#4732,.T.) ;
#6441=ORIENTED_EDGE('',*,*,#4615,.F.) ;
#6442=ORIENTED_EDGE('',*,*,#4734,.T.) ;
#6443=ORIENTED_EDGE('',*,*,#4735,.T.) ;
#6444=ORIENTED_EDGE('',*,*,#4618,.F.) ;
#6445=ORIENTED_EDGE('',*,*,#4736,.T.) ;
#6446=ORIENTED_EDGE('',*,*,#4619,.F.) ;
#6447=ORIENTED_EDGE('',*,*,#4737,.F.) ;
#6448=ORIENTED_EDGE('',*,*,#4620,.F.) ;
#6449=ORIENTED_EDGE('',*,*,#4736,.F.) ;
#6450=ORIENTED_EDGE('',*,*,#4617,.F.) ;
#6451=ORIENTED_EDGE('',*,*,#4737,.T.) ;
#6452=ORIENTED_EDGE('',*,*,#4622,.F.) ;
#6453=ORIENTED_EDGE('',*,*,#4738,.T.) ;
#6454=ORIENTED_EDGE('',*,*,#4623,.F.) ;
#6455=ORIENTED_EDGE('',*,*,#4739,.F.) ;
#6456=ORIENTED_EDGE('',*,*,#4624,.F.) ;
#6457=ORIENTED_EDGE('',*,*,#4738,.F.) ;
#6458=ORIENTED_EDGE('',*,*,#4621,.F.) ;
#6459=ORIENTED_EDGE('',*,*,#4739,.T.) ;
#6460=ORIENTED_EDGE('',*,*,#4626,.F.) ;
#6461=ORIENTED_EDGE('',*,*,#4740,.T.) ;
#6462=ORIENTED_EDGE('',*,*,#4627,.F.) ;
#6463=ORIENTED_EDGE('',*,*,#4741,.F.) ;
#6464=ORIENTED_EDGE('',*,*,#4628,.F.) ;
#6465=ORIENTED_EDGE('',*,*,#4740,.F.) ;
#6466=ORIENTED_EDGE('',*,*,#4625,.F.) ;
#6467=ORIENTED_EDGE('',*,*,#4741,.T.) ;
#6468=ORIENTED_EDGE('',*,*,#4630,.F.) ;
#6469=ORIENTED_EDGE('',*,*,#4742,.T.) ;
#6470=ORIENTED_EDGE('',*,*,#4631,.F.) ;
#6471=ORIENTED_EDGE('',*,*,#4743,.F.) ;
#6472=ORIENTED_EDGE('',*,*,#4744,.F.) ;
#6473=ORIENTED_EDGE('',*,*,#4632,.F.) ;
#6474=ORIENTED_EDGE('',*,*,#4742,.F.) ;
#6475=ORIENTED_EDGE('',*,*,#4629,.F.) ;
#6476=ORIENTED_EDGE('',*,*,#4744,.T.) ;
#6477=ORIENTED_EDGE('',*,*,#4745,.T.) ;
#6478=ORIENTED_EDGE('',*,*,#4746,.F.) ;
#6479=ORIENTED_EDGE('',*,*,#4747,.F.) ;
#6480=ORIENTED_EDGE('',*,*,#4634,.F.) ;
#6481=ORIENTED_EDGE('',*,*,#4748,.F.) ;
#6482=ORIENTED_EDGE('',*,*,#4745,.F.) ;
#6483=ORIENTED_EDGE('',*,*,#4743,.T.) ;
#6484=ORIENTED_EDGE('',*,*,#4633,.F.) ;
#6485=ORIENTED_EDGE('',*,*,#4747,.T.) ;
#6486=ORIENTED_EDGE('',*,*,#4749,.T.) ;
#6487=ORIENTED_EDGE('',*,*,#4750,.F.) ;
#6488=ORIENTED_EDGE('',*,*,#4749,.F.) ;
#6489=ORIENTED_EDGE('',*,*,#4746,.T.) ;
#6490=ORIENTED_EDGE('',*,*,#4748,.T.) ;
#6491=ORIENTED_EDGE('',*,*,#4635,.F.) ;
#6492=ORIENTED_EDGE('',*,*,#4750,.T.) ;
#7658=PLANE('',#9207) ;
#7659=PLANE('',#9318) ;
#7941=ADVANCED_FACE('',(#1554),#198,.T.) ;
#7942=ADVANCED_FACE('',(#1555),#199,.T.) ;
#7943=ADVANCED_FACE('',(#1556),#200,.T.) ;
#7944=ADVANCED_FACE('',(#1557),#201,.T.) ;
#7945=ADVANCED_FACE('',(#1558),#202,.T.) ;
#7946=ADVANCED_FACE('',(#1559),#203,.T.) ;
#7947=ADVANCED_FACE('',(#1560),#204,.T.) ;
#7948=ADVANCED_FACE('',(#1561),#205,.T.) ;
#7949=ADVANCED_FACE('',(#1562),#206,.T.) ;
#7950=ADVANCED_FACE('',(#1563),#207,.T.) ;
#7951=ADVANCED_FACE('',(#1564),#208,.T.) ;
#7952=ADVANCED_FACE('',(#1565),#209,.T.) ;
#7953=ADVANCED_FACE('',(#1566),#210,.T.) ;
#7954=ADVANCED_FACE('',(#1567),#211,.T.) ;
#7955=ADVANCED_FACE('',(#1568),#212,.T.) ;
#7956=ADVANCED_FACE('',(#1569),#213,.T.) ;
#7957=ADVANCED_FACE('',(#1570),#214,.T.) ;
#7958=ADVANCED_FACE('',(#1571),#215,.T.) ;
#7959=ADVANCED_FACE('',(#1572),#216,.T.) ;
#7960=ADVANCED_FACE('',(#1573),#217,.T.) ;
#7961=ADVANCED_FACE('',(#1574),#218,.T.) ;
#7962=ADVANCED_FACE('',(#1575),#219,.T.) ;
#7963=ADVANCED_FACE('',(#1576),#220,.T.) ;
#7964=ADVANCED_FACE('',(#1577),#221,.T.) ;
#7965=ADVANCED_FACE('',(#1578),#222,.T.) ;
#7966=ADVANCED_FACE('',(#1579),#223,.T.) ;
#7967=ADVANCED_FACE('',(#1580),#224,.T.) ;
#7968=ADVANCED_FACE('',(#1581),#225,.T.) ;
#7969=ADVANCED_FACE('',(#1582),#226,.T.) ;
#7970=ADVANCED_FACE('',(#1583),#227,.T.) ;
#7971=ADVANCED_FACE('',(#1584),#228,.T.) ;
#7972=ADVANCED_FACE('',(#1585),#229,.T.) ;
#7973=ADVANCED_FACE('',(#1586),#230,.T.) ;
#7974=ADVANCED_FACE('',(#1587),#231,.T.) ;
#7975=ADVANCED_FACE('',(#1588),#232,.T.) ;
#7976=ADVANCED_FACE('',(#1589),#233,.T.) ;
#7977=ADVANCED_FACE('',(#1590),#234,.T.) ;
#7978=ADVANCED_FACE('',(#1591),#235,.T.) ;
#7979=ADVANCED_FACE('',(#1592),#236,.T.) ;
#7980=ADVANCED_FACE('',(#1593),#688,.T.) ;
#7981=ADVANCED_FACE('',(#1594),#7658,.T.) ;
#7982=ADVANCED_FACE('',(#1595),#689,.T.) ;
#7983=ADVANCED_FACE('',(#1596),#690,.T.) ;
#7984=ADVANCED_FACE('',(#1597),#691,.T.) ;
#7985=ADVANCED_FACE('',(#1598),#692,.T.) ;
#7986=ADVANCED_FACE('',(#1599),#693,.T.) ;
#7987=ADVANCED_FACE('',(#1600),#694,.T.) ;
#7988=ADVANCED_FACE('',(#1601),#695,.T.) ;
#7989=ADVANCED_FACE('',(#1602),#696,.T.) ;
#7990=ADVANCED_FACE('',(#1603),#697,.T.) ;
#7991=ADVANCED_FACE('',(#1604),#698,.T.) ;
#7992=ADVANCED_FACE('',(#1605),#699,.T.) ;
#7993=ADVANCED_FACE('',(#1606),#700,.T.) ;
#7994=ADVANCED_FACE('',(#1607),#701,.T.) ;
#7995=ADVANCED_FACE('',(#1608),#702,.T.) ;
#7996=ADVANCED_FACE('',(#1609),#703,.T.) ;
#7997=ADVANCED_FACE('',(#1610),#704,.T.) ;
#7998=ADVANCED_FACE('',(#1611),#705,.T.) ;
#7999=ADVANCED_FACE('',(#1612),#706,.T.) ;
#8000=ADVANCED_FACE('',(#1613),#707,.T.) ;
#8001=ADVANCED_FACE('',(#1614),#708,.T.) ;
#8002=ADVANCED_FACE('',(#1615),#709,.T.) ;
#8003=ADVANCED_FACE('',(#1616),#710,.T.) ;
#8004=ADVANCED_FACE('',(#1617),#711,.T.) ;
#8005=ADVANCED_FACE('',(#1618),#712,.T.) ;
#8006=ADVANCED_FACE('',(#1619),#713,.T.) ;
#8007=ADVANCED_FACE('',(#1620),#714,.T.) ;
#8008=ADVANCED_FACE('',(#1621),#715,.T.) ;
#8009=ADVANCED_FACE('',(#1622),#716,.T.) ;
#8010=ADVANCED_FACE('',(#1623),#717,.T.) ;
#8011=ADVANCED_FACE('',(#1624),#718,.T.) ;
#8012=ADVANCED_FACE('',(#1625),#719,.T.) ;
#8013=ADVANCED_FACE('',(#1626),#720,.T.) ;
#8014=ADVANCED_FACE('',(#1627),#721,.T.) ;
#8015=ADVANCED_FACE('',(#1628),#722,.T.) ;
#8016=ADVANCED_FACE('',(#1629),#723,.T.) ;
#8017=ADVANCED_FACE('',(#1630),#724,.T.) ;
#8018=ADVANCED_FACE('',(#1631),#725,.T.) ;
#8019=ADVANCED_FACE('',(#1632),#726,.T.) ;
#8020=ADVANCED_FACE('',(#1633),#727,.T.) ;
#8021=ADVANCED_FACE('',(#1634),#7659,.T.) ;
#8271=CLOSED_SHELL('',(#7941,#7942,#7943,#7944,#7945,#7946,#7947,#7948,
#7949,#7950,#7951,#7952,#7953,#7954,#7955,#7956,#7957,#7958,#7959,#7960,
#7961,#7962,#7963,#7964,#7965,#7966,#7967,#7968,#7969,#7970,#7971,#7972,
#7973,#7974,#7975,#7976,#7977,#7978,#7979,#7980,#7981,#7982,#7983,#7984,
#7985,#7986,#7987,#7988,#7989,#7990,#7991,#7992,#7993,#7994,#7995,#7996,
#7997,#7998,#7999,#8000,#8001,#8002,#8003,#8004,#8005,#8006,#8007,#8008,
#8009,#8010,#8011,#8012,#8013,#8014,#8015,#8016,#8017,#8018,#8019,#8020,
#8021)) ;
#9044=AXIS2_PLACEMENT_3D('',#13783,#10888,#10889) ;
#9045=AXIS2_PLACEMENT_3D('',#13784,#10890,#10891) ;
#9046=AXIS2_PLACEMENT_3D('',#13787,#10892,#10893) ;
#9047=AXIS2_PLACEMENT_3D('',#13788,#10894,#10895) ;
#9048=AXIS2_PLACEMENT_3D('',#13789,#10896,#10897) ;
#9049=AXIS2_PLACEMENT_3D('',#13792,#10898,#10899) ;
#9050=AXIS2_PLACEMENT_3D('',#13794,#10900,#10901) ;
#9051=AXIS2_PLACEMENT_3D('',#13795,#10902,#10903) ;
#9052=AXIS2_PLACEMENT_3D('',#13796,#10904,#10905) ;
#9053=AXIS2_PLACEMENT_3D('',#13799,#10906,#10907) ;
#9054=AXIS2_PLACEMENT_3D('',#13801,#10908,#10909) ;
#9055=AXIS2_PLACEMENT_3D('',#13803,#10910,#10911) ;
#9056=AXIS2_PLACEMENT_3D('',#13804,#10912,#10913) ;
#9057=AXIS2_PLACEMENT_3D('',#13805,#10914,#10915) ;
#9058=AXIS2_PLACEMENT_3D('',#13808,#10916,#10917) ;
#9059=AXIS2_PLACEMENT_3D('',#13810,#10918,#10919) ;
#9060=AXIS2_PLACEMENT_3D('',#13812,#10920,#10921) ;
#9061=AXIS2_PLACEMENT_3D('',#13813,#10922,#10923) ;
#9062=AXIS2_PLACEMENT_3D('',#13814,#10924,#10925) ;
#9063=AXIS2_PLACEMENT_3D('',#13817,#10926,#10927) ;
#9064=AXIS2_PLACEMENT_3D('',#13819,#10928,#10929) ;
#9065=AXIS2_PLACEMENT_3D('',#13821,#10930,#10931) ;
#9066=AXIS2_PLACEMENT_3D('',#13822,#10932,#10933) ;
#9067=AXIS2_PLACEMENT_3D('',#13823,#10934,#10935) ;
#9068=AXIS2_PLACEMENT_3D('',#13826,#10936,#10937) ;
#9069=AXIS2_PLACEMENT_3D('',#13828,#10938,#10939) ;
#9070=AXIS2_PLACEMENT_3D('',#13829,#10940,#10941) ;
#9071=AXIS2_PLACEMENT_3D('',#13830,#10942,#10943) ;
#9072=AXIS2_PLACEMENT_3D('',#13833,#10944,#10945) ;
#9073=AXIS2_PLACEMENT_3D('',#13834,#10946,#10947) ;
#9074=AXIS2_PLACEMENT_3D('',#13835,#10948,#10949) ;
#9075=AXIS2_PLACEMENT_3D('',#13838,#10950,#10951) ;
#9076=AXIS2_PLACEMENT_3D('',#13839,#10952,#10953) ;
#9077=AXIS2_PLACEMENT_3D('',#13840,#10954,#10955) ;
#9078=AXIS2_PLACEMENT_3D('',#13843,#10956,#10957) ;
#9079=AXIS2_PLACEMENT_3D('',#13844,#10958,#10959) ;
#9080=AXIS2_PLACEMENT_3D('',#13845,#10960,#10961) ;
#9081=AXIS2_PLACEMENT_3D('',#13848,#10962,#10963) ;
#9082=AXIS2_PLACEMENT_3D('',#13850,#10964,#10965) ;
#9083=AXIS2_PLACEMENT_3D('',#13851,#10966,#10967) ;
#9084=AXIS2_PLACEMENT_3D('',#13852,#10968,#10969) ;
#9085=AXIS2_PLACEMENT_3D('',#13855,#10970,#10971) ;
#9086=AXIS2_PLACEMENT_3D('',#13857,#10972,#10973) ;
#9087=AXIS2_PLACEMENT_3D('',#13859,#10974,#10975) ;
#9088=AXIS2_PLACEMENT_3D('',#13860,#10976,#10977) ;
#9089=AXIS2_PLACEMENT_3D('',#13861,#10978,#10979) ;
#9090=AXIS2_PLACEMENT_3D('',#13864,#10980,#10981) ;
#9091=AXIS2_PLACEMENT_3D('',#13866,#10982,#10983) ;
#9092=AXIS2_PLACEMENT_3D('',#13868,#10984,#10985) ;
#9093=AXIS2_PLACEMENT_3D('',#13869,#10986,#10987) ;
#9094=AXIS2_PLACEMENT_3D('',#13870,#10988,#10989) ;
#9095=AXIS2_PLACEMENT_3D('',#13873,#10990,#10991) ;
#9096=AXIS2_PLACEMENT_3D('',#13875,#10992,#10993) ;
#9097=AXIS2_PLACEMENT_3D('',#13877,#10994,#10995) ;
#9098=AXIS2_PLACEMENT_3D('',#13878,#10996,#10997) ;
#9099=AXIS2_PLACEMENT_3D('',#13879,#10998,#10999) ;
#9100=AXIS2_PLACEMENT_3D('',#13882,#11000,#11001) ;
#9101=AXIS2_PLACEMENT_3D('',#13884,#11002,#11003) ;
#9102=AXIS2_PLACEMENT_3D('',#13885,#11004,#11005) ;
#9103=AXIS2_PLACEMENT_3D('',#13886,#11006,#11007) ;
#9104=AXIS2_PLACEMENT_3D('',#13889,#11008,#11009) ;
#9105=AXIS2_PLACEMENT_3D('',#13890,#11010,#11011) ;
#9106=AXIS2_PLACEMENT_3D('',#13891,#11012,#11013) ;
#9107=AXIS2_PLACEMENT_3D('',#13894,#11014,#11015) ;
#9108=AXIS2_PLACEMENT_3D('',#13895,#11016,#11017) ;
#9109=AXIS2_PLACEMENT_3D('',#13896,#11018,#11019) ;
#9110=AXIS2_PLACEMENT_3D('',#13899,#11020,#11021) ;
#9111=AXIS2_PLACEMENT_3D('',#13900,#11022,#11023) ;
#9112=AXIS2_PLACEMENT_3D('',#13901,#11024,#11025) ;
#9113=AXIS2_PLACEMENT_3D('',#13904,#11026,#11027) ;
#9114=AXIS2_PLACEMENT_3D('',#13906,#11028,#11029) ;
#9115=AXIS2_PLACEMENT_3D('',#13907,#11030,#11031) ;
#9116=AXIS2_PLACEMENT_3D('',#13908,#11032,#11033) ;
#9117=AXIS2_PLACEMENT_3D('',#13911,#11034,#11035) ;
#9118=AXIS2_PLACEMENT_3D('',#13913,#11036,#11037) ;
#9119=AXIS2_PLACEMENT_3D('',#13915,#11038,#11039) ;
#9120=AXIS2_PLACEMENT_3D('',#13916,#11040,#11041) ;
#9121=AXIS2_PLACEMENT_3D('',#13917,#11042,#11043) ;
#9122=AXIS2_PLACEMENT_3D('',#13920,#11044,#11045) ;
#9123=AXIS2_PLACEMENT_3D('',#13922,#11046,#11047) ;
#9124=AXIS2_PLACEMENT_3D('',#13924,#11048,#11049) ;
#9125=AXIS2_PLACEMENT_3D('',#13925,#11050,#11051) ;
#9126=AXIS2_PLACEMENT_3D('',#13926,#11052,#11053) ;
#9127=AXIS2_PLACEMENT_3D('',#13929,#11054,#11055) ;
#9128=AXIS2_PLACEMENT_3D('',#13931,#11056,#11057) ;
#9129=AXIS2_PLACEMENT_3D('',#13933,#11058,#11059) ;
#9130=AXIS2_PLACEMENT_3D('',#13934,#11060,#11061) ;
#9131=AXIS2_PLACEMENT_3D('',#13935,#11062,#11063) ;
#9132=AXIS2_PLACEMENT_3D('',#13938,#11064,#11065) ;
#9133=AXIS2_PLACEMENT_3D('',#13940,#11066,#11067) ;
#9134=AXIS2_PLACEMENT_3D('',#13941,#11068,#11069) ;
#9135=AXIS2_PLACEMENT_3D('',#13942,#11070,#11071) ;
#9136=AXIS2_PLACEMENT_3D('',#13945,#11072,#11073) ;
#9137=AXIS2_PLACEMENT_3D('',#13946,#11074,#11075) ;
#9138=AXIS2_PLACEMENT_3D('',#13947,#11076,#11077) ;
#9139=AXIS2_PLACEMENT_3D('',#13950,#11078,#11079) ;
#9140=AXIS2_PLACEMENT_3D('',#13951,#11080,#11081) ;
#9141=AXIS2_PLACEMENT_3D('',#13952,#11082,#11083) ;
#9142=AXIS2_PLACEMENT_3D('',#13955,#11084,#11085) ;
#9143=AXIS2_PLACEMENT_3D('',#13956,#11086,#11087) ;
#9144=AXIS2_PLACEMENT_3D('',#13957,#11088,#11089) ;
#9145=AXIS2_PLACEMENT_3D('',#13960,#11090,#11091) ;
#9146=AXIS2_PLACEMENT_3D('',#13962,#11092,#11093) ;
#9147=AXIS2_PLACEMENT_3D('',#13963,#11094,#11095) ;
#9148=AXIS2_PLACEMENT_3D('',#13964,#11096,#11097) ;
#9149=AXIS2_PLACEMENT_3D('',#13967,#11098,#11099) ;
#9150=AXIS2_PLACEMENT_3D('',#13969,#11100,#11101) ;
#9151=AXIS2_PLACEMENT_3D('',#13971,#11102,#11103) ;
#9152=AXIS2_PLACEMENT_3D('',#13972,#11104,#11105) ;
#9153=AXIS2_PLACEMENT_3D('',#13973,#11106,#11107) ;
#9154=AXIS2_PLACEMENT_3D('',#13976,#11108,#11109) ;
#9155=AXIS2_PLACEMENT_3D('',#13978,#11110,#11111) ;
#9156=AXIS2_PLACEMENT_3D('',#13980,#11112,#11113) ;
#9157=AXIS2_PLACEMENT_3D('',#13981,#11114,#11115) ;
#9158=AXIS2_PLACEMENT_3D('',#13982,#11116,#11117) ;
#9159=AXIS2_PLACEMENT_3D('',#13985,#11118,#11119) ;
#9160=AXIS2_PLACEMENT_3D('',#13987,#11120,#11121) ;
#9161=AXIS2_PLACEMENT_3D('',#13989,#11122,#11123) ;
#9162=AXIS2_PLACEMENT_3D('',#13990,#11124,#11125) ;
#9163=AXIS2_PLACEMENT_3D('',#13991,#11126,#11127) ;
#9164=AXIS2_PLACEMENT_3D('',#13994,#11128,#11129) ;
#9165=AXIS2_PLACEMENT_3D('',#13996,#11130,#11131) ;
#9166=AXIS2_PLACEMENT_3D('',#13997,#11132,#11133) ;
#9167=AXIS2_PLACEMENT_3D('',#13998,#11134,#11135) ;
#9168=AXIS2_PLACEMENT_3D('',#14001,#11136,#11137) ;
#9169=AXIS2_PLACEMENT_3D('',#14002,#11138,#11139) ;
#9170=AXIS2_PLACEMENT_3D('',#14003,#11140,#11141) ;
#9171=AXIS2_PLACEMENT_3D('',#14006,#11142,#11143) ;
#9172=AXIS2_PLACEMENT_3D('',#14007,#11144,#11145) ;
#9173=AXIS2_PLACEMENT_3D('',#14008,#11146,#11147) ;
#9174=AXIS2_PLACEMENT_3D('',#14011,#11148,#11149) ;
#9175=AXIS2_PLACEMENT_3D('',#14012,#11150,#11151) ;
#9176=AXIS2_PLACEMENT_3D('',#14013,#11152,#11153) ;
#9177=AXIS2_PLACEMENT_3D('',#14016,#11154,#11155) ;
#9178=AXIS2_PLACEMENT_3D('',#14018,#11156,#11157) ;
#9179=AXIS2_PLACEMENT_3D('',#14019,#11158,#11159) ;
#9180=AXIS2_PLACEMENT_3D('',#14020,#11160,#11161) ;
#9181=AXIS2_PLACEMENT_3D('',#14023,#11162,#11163) ;
#9182=AXIS2_PLACEMENT_3D('',#14025,#11164,#11165) ;
#9183=AXIS2_PLACEMENT_3D('',#14027,#11166,#11167) ;
#9184=AXIS2_PLACEMENT_3D('',#14028,#11168,#11169) ;
#9185=AXIS2_PLACEMENT_3D('',#14029,#11170,#11171) ;
#9186=AXIS2_PLACEMENT_3D('',#14032,#11172,#11173) ;
#9187=AXIS2_PLACEMENT_3D('',#14034,#11174,#11175) ;
#9188=AXIS2_PLACEMENT_3D('',#14036,#11176,#11177) ;
#9189=AXIS2_PLACEMENT_3D('',#14037,#11178,#11179) ;
#9190=AXIS2_PLACEMENT_3D('',#14038,#11180,#11181) ;
#9191=AXIS2_PLACEMENT_3D('',#14041,#11182,#11183) ;
#9192=AXIS2_PLACEMENT_3D('',#14043,#11184,#11185) ;
#9193=AXIS2_PLACEMENT_3D('',#14045,#11186,#11187) ;
#9194=AXIS2_PLACEMENT_3D('',#14046,#11188,#11189) ;
#9195=AXIS2_PLACEMENT_3D('',#14047,#11190,#11191) ;
#9196=AXIS2_PLACEMENT_3D('',#14050,#11192,#11193) ;
#9197=AXIS2_PLACEMENT_3D('',#14052,#11194,#11195) ;
#9198=AXIS2_PLACEMENT_3D('',#14053,#11196,#11197) ;
#9199=AXIS2_PLACEMENT_3D('',#14054,#11198,#11199) ;
#9200=AXIS2_PLACEMENT_3D('',#14057,#11200,#11201) ;
#9201=AXIS2_PLACEMENT_3D('',#14058,#11202,#11203) ;
#9202=AXIS2_PLACEMENT_3D('',#14059,#11204,#11205) ;
#9203=AXIS2_PLACEMENT_3D('',#14061,#11206,#11207) ;
#9204=AXIS2_PLACEMENT_3D('',#14065,#11209,#11210) ;
#9205=AXIS2_PLACEMENT_3D('',#14066,#11211,#11212) ;
#9206=AXIS2_PLACEMENT_3D('',#14067,#11213,#11214) ;
#9207=AXIS2_PLACEMENT_3D('',#14068,#11215,#11216) ;
#9208=AXIS2_PLACEMENT_3D('',#14069,#11217,#11218) ;
#9209=AXIS2_PLACEMENT_3D('',#14072,#11220,#11221) ;
#9210=AXIS2_PLACEMENT_3D('',#14073,#11222,#11223) ;
#9211=AXIS2_PLACEMENT_3D('',#14074,#11224,#11225) ;
#9212=AXIS2_PLACEMENT_3D('',#14076,#11227,#11228) ;
#9213=AXIS2_PLACEMENT_3D('',#14077,#11229,#11230) ;
#9214=AXIS2_PLACEMENT_3D('',#14079,#11232,#11233) ;
#9215=AXIS2_PLACEMENT_3D('',#14080,#11234,#11235) ;
#9216=AXIS2_PLACEMENT_3D('',#14082,#11237,#11238) ;
#9217=AXIS2_PLACEMENT_3D('',#14083,#11239,#11240) ;
#9218=AXIS2_PLACEMENT_3D('',#14086,#11242,#11243) ;
#9219=AXIS2_PLACEMENT_3D('',#14087,#11244,#11245) ;
#9220=AXIS2_PLACEMENT_3D('',#14088,#11246,#11247) ;
#9221=AXIS2_PLACEMENT_3D('',#14092,#11249,#11250) ;
#9222=AXIS2_PLACEMENT_3D('',#14093,#11251,#11252) ;
#9223=AXIS2_PLACEMENT_3D('',#14094,#11253,#11254) ;
#9224=AXIS2_PLACEMENT_3D('',#14095,#11255,#11256) ;
#9225=AXIS2_PLACEMENT_3D('',#14098,#11258,#11259) ;
#9226=AXIS2_PLACEMENT_3D('',#14099,#11260,#11261) ;
#9227=AXIS2_PLACEMENT_3D('',#14100,#11262,#11263) ;
#9228=AXIS2_PLACEMENT_3D('',#14104,#11265,#11266) ;
#9229=AXIS2_PLACEMENT_3D('',#14105,#11267,#11268) ;
#9230=AXIS2_PLACEMENT_3D('',#14106,#11269,#11270) ;
#9231=AXIS2_PLACEMENT_3D('',#14107,#11271,#11272) ;
#9232=AXIS2_PLACEMENT_3D('',#14110,#11274,#11275) ;
#9233=AXIS2_PLACEMENT_3D('',#14111,#11276,#11277) ;
#9234=AXIS2_PLACEMENT_3D('',#14112,#11278,#11279) ;
#9235=AXIS2_PLACEMENT_3D('',#14114,#11281,#11282) ;
#9236=AXIS2_PLACEMENT_3D('',#14115,#11283,#11284) ;
#9237=AXIS2_PLACEMENT_3D('',#14117,#11286,#11287) ;
#9238=AXIS2_PLACEMENT_3D('',#14118,#11288,#11289) ;
#9239=AXIS2_PLACEMENT_3D('',#14120,#11291,#11292) ;
#9240=AXIS2_PLACEMENT_3D('',#14121,#11293,#11294) ;
#9241=AXIS2_PLACEMENT_3D('',#14124,#11296,#11297) ;
#9242=AXIS2_PLACEMENT_3D('',#14125,#11298,#11299) ;
#9243=AXIS2_PLACEMENT_3D('',#14126,#11300,#11301) ;
#9244=AXIS2_PLACEMENT_3D('',#14130,#11303,#11304) ;
#9245=AXIS2_PLACEMENT_3D('',#14131,#11305,#11306) ;
#9246=AXIS2_PLACEMENT_3D('',#14132,#11307,#11308) ;
#9247=AXIS2_PLACEMENT_3D('',#14133,#11309,#11310) ;
#9248=AXIS2_PLACEMENT_3D('',#14136,#11312,#11313) ;
#9249=AXIS2_PLACEMENT_3D('',#14137,#11314,#11315) ;
#9250=AXIS2_PLACEMENT_3D('',#14138,#11316,#11317) ;
#9251=AXIS2_PLACEMENT_3D('',#14142,#11319,#11320) ;
#9252=AXIS2_PLACEMENT_3D('',#14143,#11321,#11322) ;
#9253=AXIS2_PLACEMENT_3D('',#14144,#11323,#11324) ;
#9254=AXIS2_PLACEMENT_3D('',#14145,#11325,#11326) ;
#9255=AXIS2_PLACEMENT_3D('',#14148,#11328,#11329) ;
#9256=AXIS2_PLACEMENT_3D('',#14149,#11330,#11331) ;
#9257=AXIS2_PLACEMENT_3D('',#14150,#11332,#11333) ;
#9258=AXIS2_PLACEMENT_3D('',#14152,#11335,#11336) ;
#9259=AXIS2_PLACEMENT_3D('',#14153,#11337,#11338) ;
#9260=AXIS2_PLACEMENT_3D('',#14155,#11340,#11341) ;
#9261=AXIS2_PLACEMENT_3D('',#14156,#11342,#11343) ;
#9262=AXIS2_PLACEMENT_3D('',#14158,#11345,#11346) ;
#9263=AXIS2_PLACEMENT_3D('',#14159,#11347,#11348) ;
#9264=AXIS2_PLACEMENT_3D('',#14162,#11350,#11351) ;
#9265=AXIS2_PLACEMENT_3D('',#14163,#11352,#11353) ;
#9266=AXIS2_PLACEMENT_3D('',#14164,#11354,#11355) ;
#9267=AXIS2_PLACEMENT_3D('',#14168,#11357,#11358) ;
#9268=AXIS2_PLACEMENT_3D('',#14169,#11359,#11360) ;
#9269=AXIS2_PLACEMENT_3D('',#14170,#11361,#11362) ;
#9270=AXIS2_PLACEMENT_3D('',#14171,#11363,#11364) ;
#9271=AXIS2_PLACEMENT_3D('',#14174,#11366,#11367) ;
#9272=AXIS2_PLACEMENT_3D('',#14175,#11368,#11369) ;
#9273=AXIS2_PLACEMENT_3D('',#14176,#11370,#11371) ;
#9274=AXIS2_PLACEMENT_3D('',#14180,#11373,#11374) ;
#9275=AXIS2_PLACEMENT_3D('',#14181,#11375,#11376) ;
#9276=AXIS2_PLACEMENT_3D('',#14182,#11377,#11378) ;
#9277=AXIS2_PLACEMENT_3D('',#14183,#11379,#11380) ;
#9278=AXIS2_PLACEMENT_3D('',#14186,#11382,#11383) ;
#9279=AXIS2_PLACEMENT_3D('',#14187,#11384,#11385) ;
#9280=AXIS2_PLACEMENT_3D('',#14188,#11386,#11387) ;
#9281=AXIS2_PLACEMENT_3D('',#14190,#11389,#11390) ;
#9282=AXIS2_PLACEMENT_3D('',#14191,#11391,#11392) ;
#9283=AXIS2_PLACEMENT_3D('',#14193,#11394,#11395) ;
#9284=AXIS2_PLACEMENT_3D('',#14194,#11396,#11397) ;
#9285=AXIS2_PLACEMENT_3D('',#14196,#11399,#11400) ;
#9286=AXIS2_PLACEMENT_3D('',#14197,#11401,#11402) ;
#9287=AXIS2_PLACEMENT_3D('',#14200,#11404,#11405) ;
#9288=AXIS2_PLACEMENT_3D('',#14201,#11406,#11407) ;
#9289=AXIS2_PLACEMENT_3D('',#14202,#11408,#11409) ;
#9290=AXIS2_PLACEMENT_3D('',#14206,#11411,#11412) ;
#9291=AXIS2_PLACEMENT_3D('',#14207,#11413,#11414) ;
#9292=AXIS2_PLACEMENT_3D('',#14208,#11415,#11416) ;
#9293=AXIS2_PLACEMENT_3D('',#14209,#11417,#11418) ;
#9294=AXIS2_PLACEMENT_3D('',#14212,#11420,#11421) ;
#9295=AXIS2_PLACEMENT_3D('',#14213,#11422,#11423) ;
#9296=AXIS2_PLACEMENT_3D('',#14214,#11424,#11425) ;
#9297=AXIS2_PLACEMENT_3D('',#14218,#11427,#11428) ;
#9298=AXIS2_PLACEMENT_3D('',#14219,#11429,#11430) ;
#9299=AXIS2_PLACEMENT_3D('',#14220,#11431,#11432) ;
#9300=AXIS2_PLACEMENT_3D('',#14221,#11433,#11434) ;
#9301=AXIS2_PLACEMENT_3D('',#14224,#11436,#11437) ;
#9302=AXIS2_PLACEMENT_3D('',#14225,#11438,#11439) ;
#9303=AXIS2_PLACEMENT_3D('',#14226,#11440,#11441) ;
#9304=AXIS2_PLACEMENT_3D('',#14228,#11443,#11444) ;
#9305=AXIS2_PLACEMENT_3D('',#14229,#11445,#11446) ;
#9306=AXIS2_PLACEMENT_3D('',#14231,#11448,#11449) ;
#9307=AXIS2_PLACEMENT_3D('',#14232,#11450,#11451) ;
#9308=AXIS2_PLACEMENT_3D('',#14234,#11453,#11454) ;
#9309=AXIS2_PLACEMENT_3D('',#14235,#11455,#11456) ;
#9310=AXIS2_PLACEMENT_3D('',#14238,#11458,#11459) ;
#9311=AXIS2_PLACEMENT_3D('',#14239,#11460,#11461) ;
#9312=AXIS2_PLACEMENT_3D('',#14240,#11462,#11463) ;
#9313=AXIS2_PLACEMENT_3D('',#14244,#11465,#11466) ;
#9314=AXIS2_PLACEMENT_3D('',#14245,#11467,#11468) ;
#9315=AXIS2_PLACEMENT_3D('',#14246,#11469,#11470) ;
#9316=AXIS2_PLACEMENT_3D('',#14247,#11471,#11472) ;
#9317=AXIS2_PLACEMENT_3D('',#14250,#11474,#11475) ;
#9318=AXIS2_PLACEMENT_3D('',#14251,#11476,#11477) ;
#10888=DIRECTION('axis',(0.,0.,1.)) ;
#10889=DIRECTION('refdir',(1.,0.,0.)) ;
#10890=DIRECTION('center_axis',(0.,0.,1.)) ;
#10891=DIRECTION('ref_axis',(1.,0.,0.)) ;
#10892=DIRECTION('center_axis',(-0.376865806842073,-0.909834542072809,-0.173704547103507)) ;
#10893=DIRECTION('ref_axis',(0.926267868185695,-0.370179664617619,-0.0706742687992891)) ;
#10894=DIRECTION('center_axis',(0.909834542072811,0.376865806842069,0.17370454710351)) ;
#10895=DIRECTION('ref_axis',(0.414971211111276,-0.826287510096955,-0.380851473157994)) ;
#10896=DIRECTION('center_axis',(0.,0.,1.)) ;
#10897=DIRECTION('ref_axis',(1.,0.,0.)) ;
#10898=DIRECTION('center_axis',(-0.909834542072811,-0.376865806842069,-0.17370454710351)) ;
#10899=DIRECTION('ref_axis',(0.414971211111276,-0.826287510096955,-0.380851473157994)) ;
#10900=DIRECTION('center_axis',(0.909834542072809,-0.376865806842073,0.173704547103512)) ;
#10901=DIRECTION('ref_axis',(0.41497121111128,0.826287510096954,-0.380851473157994)) ;
#10902=DIRECTION('center_axis',(0.909834542072809,-0.376865806842073,0.173704547103512)) ;
#10903=DIRECTION('ref_axis',(0.41497121111128,0.826287510096954,-0.380851473157994)) ;
#10904=DIRECTION('center_axis',(0.,0.,1.)) ;
#10905=DIRECTION('ref_axis',(-0.707106781186536,-0.707106781186559,0.)) ;
#10906=DIRECTION('center_axis',(-0.909834542072809,0.376865806842073,-0.173704547103512)) ;
#10907=DIRECTION('ref_axis',(0.41497121111128,0.826287510096954,-0.380851473157994)) ;
#10908=DIRECTION('center_axis',(-0.909834542072809,0.376865806842073,-0.173704547103512)) ;
#10909=DIRECTION('ref_axis',(0.41497121111128,0.826287510096954,-0.380851473157994)) ;
#10910=DIRECTION('center_axis',(0.376865806842071,-0.90983454207281,0.173704547103507)) ;
#10911=DIRECTION('ref_axis',(0.926267868185696,0.370179664617617,-0.0706742687992885)) ;
#10912=DIRECTION('center_axis',(0.376865806842071,-0.90983454207281,0.173704547103507)) ;
#10913=DIRECTION('ref_axis',(0.926267868185696,0.370179664617617,-0.0706742687992885)) ;
#10914=DIRECTION('center_axis',(0.,0.,1.)) ;
#10915=DIRECTION('ref_axis',(-1.,0.,0.)) ;
#10916=DIRECTION('center_axis',(-0.376865806842071,0.90983454207281,-0.173704547103507)) ;
#10917=DIRECTION('ref_axis',(0.926267868185696,0.370179664617617,-0.0706742687992885)) ;
#10918=DIRECTION('center_axis',(-0.376865806842071,0.90983454207281,-0.173704547103507)) ;
#10919=DIRECTION('ref_axis',(0.926267868185696,0.370179664617617,-0.0706742687992885)) ;
#10920=DIRECTION('center_axis',(-0.376865806842073,-0.909834542072809,0.173704547103509)) ;
#10921=DIRECTION('ref_axis',(0.926267868185696,-0.370179664617619,0.0706742687992895)) ;
#10922=DIRECTION('center_axis',(-0.376865806842073,-0.909834542072809,0.173704547103509)) ;
#10923=DIRECTION('ref_axis',(0.926267868185696,-0.370179664617619,0.0706742687992895)) ;
#10924=DIRECTION('center_axis',(0.,0.,1.)) ;
#10925=DIRECTION('ref_axis',(-0.707106781186554,0.707106781186541,0.)) ;
#10926=DIRECTION('center_axis',(0.376865806842073,0.909834542072809,-0.173704547103509)) ;
#10927=DIRECTION('ref_axis',(0.926267868185696,-0.370179664617619,0.0706742687992895)) ;
#10928=DIRECTION('center_axis',(0.376865806842073,0.909834542072809,-0.173704547103509)) ;
#10929=DIRECTION('ref_axis',(0.926267868185696,-0.370179664617619,0.0706742687992895)) ;
#10930=DIRECTION('center_axis',(-0.90983454207281,-0.376865806842072,0.173704547103508)) ;
#10931=DIRECTION('ref_axis',(0.414971211111278,-0.826287510096957,0.38085147315799)) ;
#10932=DIRECTION('center_axis',(-0.90983454207281,-0.376865806842072,0.173704547103508)) ;
#10933=DIRECTION('ref_axis',(0.414971211111278,-0.826287510096957,0.38085147315799)) ;
#10934=DIRECTION('center_axis',(0.,0.,1.)) ;
#10935=DIRECTION('ref_axis',(1.,0.,0.)) ;
#10936=DIRECTION('center_axis',(0.90983454207281,0.376865806842072,-0.173704547103508)) ;
#10937=DIRECTION('ref_axis',(0.414971211111278,-0.826287510096957,0.38085147315799)) ;
#10938=DIRECTION('center_axis',(0.90983454207281,0.376865806842072,-0.173704547103508)) ;
#10939=DIRECTION('ref_axis',(0.414971211111278,-0.826287510096957,0.38085147315799)) ;
#10940=DIRECTION('center_axis',(-0.909834542072809,0.376865806842072,0.173704547103511)) ;
#10941=DIRECTION('ref_axis',(0.414971211111279,0.826287510096954,0.380851473157994)) ;
#10942=DIRECTION('center_axis',(0.,0.,1.)) ;
#10943=DIRECTION('ref_axis',(1.,0.,0.)) ;
#10944=DIRECTION('center_axis',(0.909834542072809,-0.376865806842072,-0.173704547103511)) ;
#10945=DIRECTION('ref_axis',(0.414971211111279,0.826287510096954,0.380851473157994)) ;
#10946=DIRECTION('center_axis',(-0.376865806842072,0.909834542072809,0.17370454710351)) ;
#10947=DIRECTION('ref_axis',(0.926267868185696,0.370179664617617,0.0706742687992896)) ;
#10948=DIRECTION('center_axis',(0.,0.,1.)) ;
#10949=DIRECTION('ref_axis',(1.,0.,0.)) ;
#10950=DIRECTION('center_axis',(0.376865806842072,-0.909834542072809,-0.17370454710351)) ;
#10951=DIRECTION('ref_axis',(0.926267868185696,0.370179664617617,0.0706742687992896)) ;
#10952=DIRECTION('center_axis',(0.376865806842073,0.909834542072809,0.173704547103507)) ;
#10953=DIRECTION('ref_axis',(0.926267868185695,-0.370179664617619,-0.0706742687992891)) ;
#10954=DIRECTION('center_axis',(0.,0.,1.)) ;
#10955=DIRECTION('ref_axis',(1.,0.,0.)) ;
#10956=DIRECTION('center_axis',(-0.376865806842073,-0.909834542072809,-0.173704547103507)) ;
#10957=DIRECTION('ref_axis',(0.926267868185695,-0.370179664617619,-0.0706742687992891)) ;
#10958=DIRECTION('center_axis',(0.909834542072811,0.376865806842069,0.17370454710351)) ;
#10959=DIRECTION('ref_axis',(0.414971211111276,-0.826287510096955,-0.380851473157994)) ;
#10960=DIRECTION('center_axis',(0.,0.,1.)) ;
#10961=DIRECTION('ref_axis',(1.,0.,0.)) ;
#10962=DIRECTION('center_axis',(-0.909834542072811,-0.376865806842069,-0.17370454710351)) ;
#10963=DIRECTION('ref_axis',(0.414971211111276,-0.826287510096955,-0.380851473157994)) ;
#10964=DIRECTION('center_axis',(0.909834542072809,-0.376865806842073,0.173704547103508)) ;
#10965=DIRECTION('ref_axis',(0.414971211111279,0.826287510096957,-0.380851473157988)) ;
#10966=DIRECTION('center_axis',(0.909834542072809,-0.376865806842073,0.173704547103508)) ;
#10967=DIRECTION('ref_axis',(0.414971211111279,0.826287510096957,-0.380851473157988)) ;
#10968=DIRECTION('center_axis',(0.,0.,1.)) ;
#10969=DIRECTION('ref_axis',(-0.707106781186543,-0.707106781186552,0.)) ;
#10970=DIRECTION('center_axis',(-0.909834542072809,0.376865806842073,-0.173704547103508)) ;
#10971=DIRECTION('ref_axis',(0.414971211111279,0.826287510096957,-0.380851473157988)) ;
#10972=DIRECTION('center_axis',(-0.909834542072809,0.376865806842073,-0.173704547103508)) ;
#10973=DIRECTION('ref_axis',(0.414971211111279,0.826287510096957,-0.380851473157988)) ;
#10974=DIRECTION('center_axis',(0.376865806842071,-0.90983454207281,0.17370454710351)) ;
#10975=DIRECTION('ref_axis',(0.926267868185696,0.370179664617617,-0.0706742687992895)) ;
#10976=DIRECTION('center_axis',(0.376865806842071,-0.90983454207281,0.17370454710351)) ;
#10977=DIRECTION('ref_axis',(0.926267868185696,0.370179664617617,-0.0706742687992895)) ;
#10978=DIRECTION('center_axis',(0.,0.,1.)) ;
#10979=DIRECTION('ref_axis',(-1.,0.,0.)) ;
#10980=DIRECTION('center_axis',(-0.376865806842071,0.90983454207281,-0.17370454710351)) ;
#10981=DIRECTION('ref_axis',(0.926267868185696,0.370179664617617,-0.0706742687992895)) ;
#10982=DIRECTION('center_axis',(-0.376865806842071,0.90983454207281,-0.17370454710351)) ;
#10983=DIRECTION('ref_axis',(0.926267868185696,0.370179664617617,-0.0706742687992895)) ;
#10984=DIRECTION('center_axis',(-0.376865806842073,-0.909834542072809,0.173704547103508)) ;
#10985=DIRECTION('ref_axis',(0.926267868185696,-0.370179664617619,0.0706742687992894)) ;
#10986=DIRECTION('center_axis',(-0.376865806842073,-0.909834542072809,0.173704547103508)) ;
#10987=DIRECTION('ref_axis',(0.926267868185696,-0.370179664617619,0.0706742687992894)) ;
#10988=DIRECTION('center_axis',(0.,0.,1.)) ;
#10989=DIRECTION('ref_axis',(-0.707106781186554,0.707106781186541,0.)) ;
#10990=DIRECTION('center_axis',(0.376865806842073,0.909834542072809,-0.173704547103508)) ;
#10991=DIRECTION('ref_axis',(0.926267868185696,-0.370179664617619,0.0706742687992894)) ;
#10992=DIRECTION('center_axis',(0.376865806842073,0.909834542072809,-0.173704547103508)) ;
#10993=DIRECTION('ref_axis',(0.926267868185696,-0.370179664617619,0.0706742687992894)) ;
#10994=DIRECTION('center_axis',(-0.909834542072809,-0.376865806842072,0.17370454710351)) ;
#10995=DIRECTION('ref_axis',(0.414971211111279,-0.826287510096955,0.380851473157994)) ;
#10996=DIRECTION('center_axis',(-0.909834542072809,-0.376865806842072,0.17370454710351)) ;
#10997=DIRECTION('ref_axis',(0.414971211111279,-0.826287510096955,0.380851473157994)) ;
#10998=DIRECTION('center_axis',(0.,0.,1.)) ;
#10999=DIRECTION('ref_axis',(1.,0.,0.)) ;
#11000=DIRECTION('center_axis',(0.909834542072809,0.376865806842072,-0.17370454710351)) ;
#11001=DIRECTION('ref_axis',(0.414971211111279,-0.826287510096955,0.380851473157994)) ;
#11002=DIRECTION('center_axis',(0.909834542072809,0.376865806842072,-0.17370454710351)) ;
#11003=DIRECTION('ref_axis',(0.414971211111279,-0.826287510096955,0.380851473157994)) ;
#11004=DIRECTION('center_axis',(-0.90983454207281,0.376865806842072,0.173704547103509)) ;
#11005=DIRECTION('ref_axis',(0.414971211111278,0.826287510096956,0.38085147315799)) ;
#11006=DIRECTION('center_axis',(0.,0.,1.)) ;
#11007=DIRECTION('ref_axis',(1.,0.,0.)) ;
#11008=DIRECTION('center_axis',(0.90983454207281,-0.376865806842072,-0.173704547103509)) ;
#11009=DIRECTION('ref_axis',(0.414971211111278,0.826287510096956,0.38085147315799)) ;
#11010=DIRECTION('center_axis',(-0.376865806842072,0.909834542072809,0.173704547103509)) ;
#11011=DIRECTION('ref_axis',(0.926267868185696,0.370179664617618,0.0706742687992892)) ;
#11012=DIRECTION('center_axis',(0.,0.,1.)) ;
#11013=DIRECTION('ref_axis',(1.,0.,0.)) ;
#11014=DIRECTION('center_axis',(0.376865806842072,-0.909834542072809,-0.173704547103509)) ;
#11015=DIRECTION('ref_axis',(0.926267868185696,0.370179664617618,0.0706742687992892)) ;
#11016=DIRECTION('center_axis',(0.376865806842073,0.909834542072809,0.173704547103509)) ;
#11017=DIRECTION('ref_axis',(0.926267868185696,-0.370179664617619,-0.0706742687992895)) ;
#11018=DIRECTION('center_axis',(0.,0.,1.)) ;
#11019=DIRECTION('ref_axis',(1.,0.,0.)) ;
#11020=DIRECTION('center_axis',(-0.376865806842073,-0.909834542072809,-0.173704547103509)) ;
#11021=DIRECTION('ref_axis',(0.926267868185696,-0.370179664617619,-0.0706742687992895)) ;
#11022=DIRECTION('center_axis',(0.90983454207281,0.37686580684207,0.173704547103509)) ;
#11023=DIRECTION('ref_axis',(0.414971211111277,-0.826287510096957,-0.380851473157992)) ;
#11024=DIRECTION('center_axis',(0.,0.,1.)) ;
#11025=DIRECTION('ref_axis',(1.,0.,0.)) ;
#11026=DIRECTION('center_axis',(-0.90983454207281,-0.37686580684207,-0.173704547103509)) ;
#11027=DIRECTION('ref_axis',(0.414971211111277,-0.826287510096957,-0.380851473157992)) ;
#11028=DIRECTION('center_axis',(0.909834542072809,-0.376865806842073,0.17370454710351)) ;
#11029=DIRECTION('ref_axis',(0.41497121111128,0.826287510096955,-0.380851473157992)) ;
#11030=DIRECTION('center_axis',(0.909834542072809,-0.376865806842073,0.17370454710351)) ;
#11031=DIRECTION('ref_axis',(0.41497121111128,0.826287510096955,-0.380851473157992)) ;
#11032=DIRECTION('center_axis',(0.,0.,1.)) ;
#11033=DIRECTION('ref_axis',(-0.707106781186556,-0.707106781186539,0.)) ;
#11034=DIRECTION('center_axis',(-0.909834542072809,0.376865806842073,-0.17370454710351)) ;
#11035=DIRECTION('ref_axis',(0.41497121111128,0.826287510096955,-0.380851473157992)) ;
#11036=DIRECTION('center_axis',(-0.909834542072809,0.376865806842073,-0.17370454710351)) ;
#11037=DIRECTION('ref_axis',(0.41497121111128,0.826287510096955,-0.380851473157992)) ;
#11038=DIRECTION('center_axis',(0.376865806842071,-0.90983454207281,0.173704547103509)) ;
#11039=DIRECTION('ref_axis',(0.926267868185696,0.370179664617617,-0.070674268799289)) ;
#11040=DIRECTION('center_axis',(0.376865806842071,-0.90983454207281,0.173704547103509)) ;
#11041=DIRECTION('ref_axis',(0.926267868185696,0.370179664617617,-0.070674268799289)) ;
#11042=DIRECTION('center_axis',(0.,0.,1.)) ;
#11043=DIRECTION('ref_axis',(-1.,2.22044604925032E-14,0.)) ;
#11044=DIRECTION('center_axis',(-0.376865806842071,0.90983454207281,-0.173704547103509)) ;
#11045=DIRECTION('ref_axis',(0.926267868185696,0.370179664617617,-0.070674268799289)) ;
#11046=DIRECTION('center_axis',(-0.376865806842071,0.90983454207281,-0.173704547103509)) ;
#11047=DIRECTION('ref_axis',(0.926267868185696,0.370179664617617,-0.070674268799289)) ;
#11048=DIRECTION('center_axis',(-0.376865806842073,-0.909834542072809,0.17370454710351)) ;
#11049=DIRECTION('ref_axis',(0.926267868185696,-0.370179664617618,0.0706742687992898)) ;
#11050=DIRECTION('center_axis',(-0.376865806842073,-0.909834542072809,0.17370454710351)) ;
#11051=DIRECTION('ref_axis',(0.926267868185696,-0.370179664617618,0.0706742687992898)) ;
#11052=DIRECTION('center_axis',(0.,0.,1.)) ;
#11053=DIRECTION('ref_axis',(-0.707106781186572,0.707106781186523,0.)) ;
#11054=DIRECTION('center_axis',(0.376865806842073,0.909834542072809,-0.17370454710351)) ;
#11055=DIRECTION('ref_axis',(0.926267868185696,-0.370179664617618,0.0706742687992898)) ;
#11056=DIRECTION('center_axis',(0.376865806842073,0.909834542072809,-0.17370454710351)) ;
#11057=DIRECTION('ref_axis',(0.926267868185696,-0.370179664617618,0.0706742687992898)) ;
#11058=DIRECTION('center_axis',(-0.90983454207281,-0.376865806842071,0.173704547103508)) ;
#11059=DIRECTION('ref_axis',(0.414971211111277,-0.826287510096957,0.38085147315799)) ;
#11060=DIRECTION('center_axis',(-0.90983454207281,-0.376865806842071,0.173704547103508)) ;
#11061=DIRECTION('ref_axis',(0.414971211111277,-0.826287510096957,0.38085147315799)) ;
#11062=DIRECTION('center_axis',(0.,0.,1.)) ;
#11063=DIRECTION('ref_axis',(1.,0.,0.)) ;
#11064=DIRECTION('center_axis',(0.90983454207281,0.376865806842071,-0.173704547103508)) ;
#11065=DIRECTION('ref_axis',(0.414971211111277,-0.826287510096957,0.38085147315799)) ;
#11066=DIRECTION('center_axis',(0.90983454207281,0.376865806842071,-0.173704547103508)) ;
#11067=DIRECTION('ref_axis',(0.414971211111277,-0.826287510096957,0.38085147315799)) ;
#11068=DIRECTION('center_axis',(-0.909834542072809,0.376865806842072,0.17370454710351)) ;
#11069=DIRECTION('ref_axis',(0.414971211111279,0.826287510096955,0.380851473157992)) ;
#11070=DIRECTION('center_axis',(0.,0.,1.)) ;
#11071=DIRECTION('ref_axis',(1.,0.,0.)) ;
#11072=DIRECTION('center_axis',(0.909834542072809,-0.376865806842072,-0.17370454710351)) ;
#11073=DIRECTION('ref_axis',(0.414971211111279,0.826287510096955,0.380851473157992)) ;
#11074=DIRECTION('center_axis',(-0.376865806842072,0.909834542072809,0.173704547103509)) ;
#11075=DIRECTION('ref_axis',(0.926267868185696,0.370179664617618,0.0706742687992893)) ;
#11076=DIRECTION('center_axis',(0.,0.,1.)) ;
#11077=DIRECTION('ref_axis',(1.,0.,0.)) ;
#11078=DIRECTION('center_axis',(0.376865806842072,-0.909834542072809,-0.173704547103509)) ;
#11079=DIRECTION('ref_axis',(0.926267868185696,0.370179664617618,0.0706742687992893)) ;
#11080=DIRECTION('center_axis',(0.376865806842073,0.909834542072809,0.17370454710351)) ;
#11081=DIRECTION('ref_axis',(0.926267868185696,-0.370179664617619,-0.0706742687992899)) ;
#11082=DIRECTION('center_axis',(0.,0.,1.)) ;
#11083=DIRECTION('ref_axis',(1.,0.,0.)) ;
#11084=DIRECTION('center_axis',(-0.376865806842073,-0.909834542072809,-0.17370454710351)) ;
#11085=DIRECTION('ref_axis',(0.926267868185696,-0.370179664617619,-0.0706742687992899)) ;
#11086=DIRECTION('center_axis',(0.90983454207281,0.376865806842072,0.173704547103509)) ;
#11087=DIRECTION('ref_axis',(0.414971211111278,-0.826287510096956,-0.380851473157991)) ;
#11088=DIRECTION('center_axis',(0.,0.,1.)) ;
#11089=DIRECTION('ref_axis',(1.,0.,0.)) ;
#11090=DIRECTION('center_axis',(-0.90983454207281,-0.376865806842072,-0.173704547103509)) ;
#11091=DIRECTION('ref_axis',(0.414971211111278,-0.826287510096956,-0.380851473157991)) ;
#11092=DIRECTION('center_axis',(0.90983454207281,-0.376865806842072,0.173704547103508)) ;
#11093=DIRECTION('ref_axis',(0.414971211111278,0.826287510096957,-0.380851473157989)) ;
#11094=DIRECTION('center_axis',(0.90983454207281,-0.376865806842072,0.173704547103508)) ;
#11095=DIRECTION('ref_axis',(0.414971211111278,0.826287510096957,-0.380851473157989)) ;
#11096=DIRECTION('center_axis',(0.,0.,1.)) ;
#11097=DIRECTION('ref_axis',(-0.707106781186543,-0.707106781186552,0.)) ;
#11098=DIRECTION('center_axis',(-0.90983454207281,0.376865806842072,-0.173704547103508)) ;
#11099=DIRECTION('ref_axis',(0.414971211111278,0.826287510096957,-0.380851473157989)) ;
#11100=DIRECTION('center_axis',(-0.90983454207281,0.376865806842072,-0.173704547103508)) ;
#11101=DIRECTION('ref_axis',(0.414971211111278,0.826287510096957,-0.380851473157989)) ;
#11102=DIRECTION('center_axis',(0.376865806842071,-0.90983454207281,0.173704547103509)) ;
#11103=DIRECTION('ref_axis',(0.926267868185696,0.370179664617617,-0.0706742687992893)) ;
#11104=DIRECTION('center_axis',(0.376865806842071,-0.90983454207281,0.173704547103509)) ;
#11105=DIRECTION('ref_axis',(0.926267868185696,0.370179664617617,-0.0706742687992893)) ;
#11106=DIRECTION('center_axis',(0.,0.,1.)) ;
#11107=DIRECTION('ref_axis',(-1.,0.,0.)) ;
#11108=DIRECTION('center_axis',(-0.376865806842071,0.90983454207281,-0.173704547103509)) ;
#11109=DIRECTION('ref_axis',(0.926267868185696,0.370179664617617,-0.0706742687992893)) ;
#11110=DIRECTION('center_axis',(-0.376865806842071,0.90983454207281,-0.173704547103509)) ;
#11111=DIRECTION('ref_axis',(0.926267868185696,0.370179664617617,-0.0706742687992893)) ;
#11112=DIRECTION('center_axis',(-0.376865806842073,-0.909834542072809,0.173704547103509)) ;
#11113=DIRECTION('ref_axis',(0.926267868185696,-0.370179664617619,0.0706742687992897)) ;
#11114=DIRECTION('center_axis',(-0.376865806842073,-0.909834542072809,0.173704547103509)) ;
#11115=DIRECTION('ref_axis',(0.926267868185696,-0.370179664617619,0.0706742687992897)) ;
#11116=DIRECTION('center_axis',(0.,0.,1.)) ;
#11117=DIRECTION('ref_axis',(-0.707106781186574,0.707106781186521,0.)) ;
#11118=DIRECTION('center_axis',(0.376865806842073,0.909834542072809,-0.173704547103509)) ;
#11119=DIRECTION('ref_axis',(0.926267868185696,-0.370179664617619,0.0706742687992897)) ;
#11120=DIRECTION('center_axis',(0.376865806842073,0.909834542072809,-0.173704547103509)) ;
#11121=DIRECTION('ref_axis',(0.926267868185696,-0.370179664617619,0.0706742687992897)) ;
#11122=DIRECTION('center_axis',(-0.90983454207281,-0.376865806842072,0.17370454710351)) ;
#11123=DIRECTION('ref_axis',(0.414971211111278,-0.826287510096955,0.380851473157992)) ;
#11124=DIRECTION('center_axis',(-0.90983454207281,-0.376865806842072,0.17370454710351)) ;
#11125=DIRECTION('ref_axis',(0.414971211111278,-0.826287510096955,0.380851473157992)) ;
#11126=DIRECTION('center_axis',(0.,0.,1.)) ;
#11127=DIRECTION('ref_axis',(1.,0.,0.)) ;
#11128=DIRECTION('center_axis',(0.90983454207281,0.376865806842072,-0.17370454710351)) ;
#11129=DIRECTION('ref_axis',(0.414971211111278,-0.826287510096955,0.380851473157992)) ;
#11130=DIRECTION('center_axis',(0.90983454207281,0.376865806842072,-0.17370454710351)) ;
#11131=DIRECTION('ref_axis',(0.414971211111278,-0.826287510096955,0.380851473157992)) ;
#11132=DIRECTION('center_axis',(-0.909834542072809,0.376865806842072,0.173704547103509)) ;
#11133=DIRECTION('ref_axis',(0.414971211111278,0.826287510096956,0.38085147315799)) ;
#11134=DIRECTION('center_axis',(0.,0.,1.)) ;
#11135=DIRECTION('ref_axis',(1.,0.,0.)) ;
#11136=DIRECTION('center_axis',(0.909834542072809,-0.376865806842072,-0.173704547103509)) ;
#11137=DIRECTION('ref_axis',(0.414971211111278,0.826287510096956,0.38085147315799)) ;
#11138=DIRECTION('center_axis',(-0.376865806842072,0.909834542072809,0.173704547103509)) ;
#11139=DIRECTION('ref_axis',(0.926267868185696,0.370179664617618,0.0706742687992893)) ;
#11140=DIRECTION('center_axis',(0.,0.,1.)) ;
#11141=DIRECTION('ref_axis',(1.,0.,0.)) ;
#11142=DIRECTION('center_axis',(0.376865806842072,-0.909834542072809,-0.173704547103509)) ;
#11143=DIRECTION('ref_axis',(0.926267868185696,0.370179664617618,0.0706742687992893)) ;
#11144=DIRECTION('center_axis',(0.376865806842073,0.909834542072809,0.173704547103509)) ;
#11145=DIRECTION('ref_axis',(0.926267868185696,-0.370179664617618,-0.0706742687992894)) ;
#11146=DIRECTION('center_axis',(0.,0.,1.)) ;
#11147=DIRECTION('ref_axis',(1.,0.,0.)) ;
#11148=DIRECTION('center_axis',(-0.376865806842073,-0.909834542072809,-0.173704547103509)) ;
#11149=DIRECTION('ref_axis',(0.926267868185696,-0.370179664617618,-0.0706742687992894)) ;
#11150=DIRECTION('center_axis',(0.909834542072809,0.376865806842072,0.173704547103509)) ;
#11151=DIRECTION('ref_axis',(0.414971211111279,-0.826287510096956,-0.380851473157991)) ;
#11152=DIRECTION('center_axis',(0.,0.,1.)) ;
#11153=DIRECTION('ref_axis',(1.,0.,0.)) ;
#11154=DIRECTION('center_axis',(-0.909834542072809,-0.376865806842072,-0.173704547103509)) ;
#11155=DIRECTION('ref_axis',(0.414971211111279,-0.826287510096956,-0.380851473157991)) ;
#11156=DIRECTION('center_axis',(0.90983454207281,-0.376865806842072,0.173704547103509)) ;
#11157=DIRECTION('ref_axis',(0.414971211111278,0.826287510096956,-0.380851473157991)) ;
#11158=DIRECTION('center_axis',(0.90983454207281,-0.376865806842072,0.173704547103509)) ;
#11159=DIRECTION('ref_axis',(0.414971211111278,0.826287510096956,-0.380851473157991)) ;
#11160=DIRECTION('center_axis',(0.,0.,1.)) ;
#11161=DIRECTION('ref_axis',(-0.707106781186572,-0.707106781186523,0.)) ;
#11162=DIRECTION('center_axis',(-0.90983454207281,0.376865806842072,-0.173704547103509)) ;
#11163=DIRECTION('ref_axis',(0.414971211111278,0.826287510096956,-0.380851473157991)) ;
#11164=DIRECTION('center_axis',(-0.90983454207281,0.376865806842072,-0.173704547103509)) ;
#11165=DIRECTION('ref_axis',(0.414971211111278,0.826287510096956,-0.380851473157991)) ;
#11166=DIRECTION('center_axis',(0.376865806842071,-0.90983454207281,0.173704547103509)) ;
#11167=DIRECTION('ref_axis',(0.926267868185696,0.370179664617617,-0.0706742687992893)) ;
#11168=DIRECTION('center_axis',(0.376865806842071,-0.90983454207281,0.173704547103509)) ;
#11169=DIRECTION('ref_axis',(0.926267868185696,0.370179664617617,-0.0706742687992893)) ;
#11170=DIRECTION('center_axis',(0.,0.,1.)) ;
#11171=DIRECTION('ref_axis',(-1.,0.,0.)) ;
#11172=DIRECTION('center_axis',(-0.376865806842071,0.90983454207281,-0.173704547103509)) ;
#11173=DIRECTION('ref_axis',(0.926267868185696,0.370179664617617,-0.0706742687992893)) ;
#11174=DIRECTION('center_axis',(-0.376865806842071,0.90983454207281,-0.173704547103509)) ;
#11175=DIRECTION('ref_axis',(0.926267868185696,0.370179664617617,-0.0706742687992893)) ;
#11176=DIRECTION('center_axis',(-0.376865806842072,-0.90983454207281,0.173704547103509)) ;
#11177=DIRECTION('ref_axis',(0.926267868185696,-0.370179664617617,0.0706742687992892)) ;
#11178=DIRECTION('center_axis',(-0.376865806842072,-0.90983454207281,0.173704547103509)) ;
#11179=DIRECTION('ref_axis',(0.926267868185696,-0.370179664617617,0.0706742687992892)) ;
#11180=DIRECTION('center_axis',(0.,0.,1.)) ;
#11181=DIRECTION('ref_axis',(-0.707106781186561,0.707106781186534,0.)) ;
#11182=DIRECTION('center_axis',(0.376865806842072,0.90983454207281,-0.173704547103509)) ;
#11183=DIRECTION('ref_axis',(0.926267868185696,-0.370179664617617,0.0706742687992892)) ;
#11184=DIRECTION('center_axis',(0.376865806842072,0.90983454207281,-0.173704547103509)) ;
#11185=DIRECTION('ref_axis',(0.926267868185696,-0.370179664617617,0.0706742687992892)) ;
#11186=DIRECTION('center_axis',(-0.90983454207281,-0.376865806842072,0.173704547103509)) ;
#11187=DIRECTION('ref_axis',(0.414971211111278,-0.826287510096956,0.380851473157991)) ;
#11188=DIRECTION('center_axis',(-0.90983454207281,-0.376865806842072,0.173704547103509)) ;
#11189=DIRECTION('ref_axis',(0.414971211111278,-0.826287510096956,0.380851473157991)) ;
#11190=DIRECTION('center_axis',(0.,0.,1.)) ;
#11191=DIRECTION('ref_axis',(1.,0.,0.)) ;
#11192=DIRECTION('center_axis',(0.90983454207281,0.376865806842072,-0.173704547103509)) ;
#11193=DIRECTION('ref_axis',(0.414971211111278,-0.826287510096956,0.380851473157991)) ;
#11194=DIRECTION('center_axis',(0.90983454207281,0.376865806842072,-0.173704547103509)) ;
#11195=DIRECTION('ref_axis',(0.414971211111278,-0.826287510096956,0.380851473157991)) ;
#11196=DIRECTION('center_axis',(-0.909834542072809,0.376865806842072,0.173704547103509)) ;
#11197=DIRECTION('ref_axis',(0.414971211111278,0.826287510096956,0.38085147315799)) ;
#11198=DIRECTION('center_axis',(0.,0.,1.)) ;
#11199=DIRECTION('ref_axis',(1.,0.,0.)) ;
#11200=DIRECTION('center_axis',(0.909834542072809,-0.376865806842072,-0.173704547103509)) ;
#11201=DIRECTION('ref_axis',(0.414971211111278,0.826287510096956,0.38085147315799)) ;
#11202=DIRECTION('center_axis',(-0.376865806842073,0.909834542072809,0.173704547103509)) ;
#11203=DIRECTION('ref_axis',(0.926267868185696,0.370179664617618,0.0706742687992896)) ;
#11204=DIRECTION('center_axis',(0.376865806842073,0.909834542072809,0.173704547103507)) ;
#11205=DIRECTION('ref_axis',(0.926267868185695,-0.370179664617619,-0.0706742687992891)) ;
#11206=DIRECTION('center_axis',(0.376865806842073,0.909834542072809,0.173704547103507)) ;
#11207=DIRECTION('ref_axis',(0.926267868185695,-0.370179664617619,-0.0706742687992891)) ;
#11208=DIRECTION('',(-0.376865806842074,-0.909834542072809,-0.173704547103507)) ;
#11209=DIRECTION('center_axis',(-0.694561688421286,-0.694561688421282,-0.187531655873747)) ;
#11210=DIRECTION('ref_axis',(0.707106781186545,-0.70710678118655,4.46695575243751E-15)) ;
#11211=DIRECTION('center_axis',(-0.694561688421286,-0.694561688421282,-0.187531655873747)) ;
#11212=DIRECTION('ref_axis',(0.707106781186545,-0.70710678118655,4.46695575243751E-15)) ;
#11213=DIRECTION('center_axis',(-0.694561688421286,-0.694561688421282,-0.187531655873747)) ;
#11214=DIRECTION('ref_axis',(0.707106781186545,-0.70710678118655,4.46695575243751E-15)) ;
#11215=DIRECTION('center_axis',(0.376865806842073,0.909834542072809,0.173704547103507)) ;
#11216=DIRECTION('ref_axis',(0.926267868185696,-0.370179664617619,-0.0706742687992891)) ;
#11217=DIRECTION('center_axis',(0.909834542072811,0.376865806842069,0.17370454710351)) ;
#11218=DIRECTION('ref_axis',(0.414971211111276,-0.826287510096955,-0.380851473157994)) ;
#11219=DIRECTION('',(-0.909834542072811,-0.376865806842069,-0.17370454710351)) ;
#11220=DIRECTION('center_axis',(-0.982258559670136,9.62376035907939E-15,
-0.187531655873751)) ;
#11221=DIRECTION('ref_axis',(-1.14405485458112E-14,-1.,8.16263856920234E-15)) ;
#11222=DIRECTION('center_axis',(-0.982258559670136,9.62376035907939E-15,
-0.187531655873751)) ;
#11223=DIRECTION('ref_axis',(-1.14405485458112E-14,-1.,8.16263856920234E-15)) ;
#11224=DIRECTION('center_axis',(0.909834542072809,-0.376865806842073,0.173704547103512)) ;
#11225=DIRECTION('ref_axis',(0.41497121111128,0.826287510096954,-0.380851473157994)) ;
#11226=DIRECTION('',(-0.909834542072809,0.376865806842073,-0.173704547103512)) ;
#11227=DIRECTION('center_axis',(-0.694561688421282,0.694561688421288,-0.187531655873744)) ;
#11228=DIRECTION('ref_axis',(0.707106781186549,0.707106781186546,1.52005041072154E-14)) ;
#11229=DIRECTION('center_axis',(0.376865806842071,-0.90983454207281,0.173704547103507)) ;
#11230=DIRECTION('ref_axis',(0.926267868185696,0.370179664617617,-0.0706742687992885)) ;
#11231=DIRECTION('',(-0.376865806842071,0.90983454207281,-0.173704547103507)) ;
#11232=DIRECTION('center_axis',(5.58328333024527E-15,0.982258559670136,
-0.187531655873747)) ;
#11233=DIRECTION('ref_axis',(1.,-5.52745603898742E-15,1.06050028654991E-15)) ;
#11234=DIRECTION('center_axis',(-0.376865806842073,-0.909834542072809,0.173704547103509)) ;
#11235=DIRECTION('ref_axis',(0.926267868185696,-0.370179664617619,0.0706742687992895)) ;
#11236=DIRECTION('',(0.376865806842073,0.909834542072809,-0.173704547103509)) ;
#11237=DIRECTION('center_axis',(0.694561688421279,0.69456168842129,-0.187531655873747)) ;
#11238=DIRECTION('ref_axis',(0.707106781186552,-0.707106781186543,-3.03688718421113E-15)) ;
#11239=DIRECTION('center_axis',(-0.90983454207281,-0.376865806842072,0.173704547103508)) ;
#11240=DIRECTION('ref_axis',(0.414971211111278,-0.826287510096957,0.38085147315799)) ;
#11241=DIRECTION('',(0.90983454207281,0.376865806842072,-0.173704547103508)) ;
#11242=DIRECTION('center_axis',(0.982258559670136,6.5381477562569E-15,-0.187531655873751)) ;
#11243=DIRECTION('ref_axis',(3.85636467836333E-15,-1.,-1.43970947992231E-14)) ;
#11244=DIRECTION('center_axis',(0.982258559670136,6.5381477562569E-15,-0.187531655873751)) ;
#11245=DIRECTION('ref_axis',(3.85636467836333E-15,-1.,-1.43970947992231E-14)) ;
#11246=DIRECTION('center_axis',(-0.909834542072809,0.376865806842072,0.173704547103511)) ;
#11247=DIRECTION('ref_axis',(0.414971211111279,0.826287510096954,0.380851473157994)) ;
#11248=DIRECTION('',(0.909834542072809,-0.376865806842072,-0.173704547103511)) ;
#11249=DIRECTION('center_axis',(0.69456168842128,-0.694561688421288,-0.187531655873747)) ;
#11250=DIRECTION('ref_axis',(0.707106781186551,0.707106781186544,-5.65600152826619E-15)) ;
#11251=DIRECTION('center_axis',(0.69456168842128,-0.694561688421288,-0.187531655873747)) ;
#11252=DIRECTION('ref_axis',(0.707106781186551,0.707106781186544,-5.65600152826619E-15)) ;
#11253=DIRECTION('center_axis',(0.69456168842128,-0.694561688421288,-0.187531655873747)) ;
#11254=DIRECTION('ref_axis',(0.707106781186551,0.707106781186544,-5.65600152826619E-15)) ;
#11255=DIRECTION('center_axis',(-0.376865806842072,0.909834542072809,0.17370454710351)) ;
#11256=DIRECTION('ref_axis',(0.926267868185696,0.370179664617617,0.0706742687992896)) ;
#11257=DIRECTION('',(0.376865806842072,-0.909834542072809,-0.17370454710351)) ;
#11258=DIRECTION('center_axis',(-4.0404770288341E-15,-0.982258559670136,
-0.187531655873747)) ;
#11259=DIRECTION('ref_axis',(1.,-3.98491016764209E-15,-7.79307028752587E-16)) ;
#11260=DIRECTION('center_axis',(-4.0404770288341E-15,-0.982258559670136,
-0.187531655873747)) ;
#11261=DIRECTION('ref_axis',(1.,-3.98491016764209E-15,-7.79307028752587E-16)) ;
#11262=DIRECTION('center_axis',(0.376865806842073,0.909834542072809,0.173704547103507)) ;
#11263=DIRECTION('ref_axis',(0.926267868185695,-0.370179664617619,-0.0706742687992891)) ;
#11264=DIRECTION('',(-0.376865806842073,-0.909834542072809,-0.173704547103507)) ;
#11265=DIRECTION('center_axis',(-0.694561688421286,-0.694561688421282,-0.187531655873747)) ;
#11266=DIRECTION('ref_axis',(0.707106781186545,-0.70710678118655,4.46695575243751E-15)) ;
#11267=DIRECTION('center_axis',(-0.694561688421286,-0.694561688421282,-0.187531655873747)) ;
#11268=DIRECTION('ref_axis',(0.707106781186545,-0.70710678118655,4.46695575243751E-15)) ;
#11269=DIRECTION('center_axis',(-0.694561688421286,-0.694561688421282,-0.187531655873747)) ;
#11270=DIRECTION('ref_axis',(0.707106781186545,-0.70710678118655,4.46695575243751E-15)) ;
#11271=DIRECTION('center_axis',(0.909834542072811,0.376865806842069,0.17370454710351)) ;
#11272=DIRECTION('ref_axis',(0.414971211111276,-0.826287510096955,-0.380851473157994)) ;
#11273=DIRECTION('',(-0.909834542072811,-0.376865806842069,-0.17370454710351)) ;
#11274=DIRECTION('center_axis',(-0.982258559670137,6.53814775625699E-15,
-0.187531655873742)) ;
#11275=DIRECTION('ref_axis',(-4.2259329600398E-15,-1.,-1.29188216725171E-14)) ;
#11276=DIRECTION('center_axis',(-0.982258559670137,6.53814775625699E-15,
-0.187531655873742)) ;
#11277=DIRECTION('ref_axis',(-4.2259329600398E-15,-1.,-1.29188216725171E-14)) ;
#11278=DIRECTION('center_axis',(0.909834542072809,-0.376865806842073,0.173704547103508)) ;
#11279=DIRECTION('ref_axis',(0.414971211111279,0.826287510096957,-0.380851473157988)) ;
#11280=DIRECTION('',(-0.909834542072809,0.376865806842073,-0.173704547103508)) ;
#11281=DIRECTION('center_axis',(-0.694561688421284,0.694561688421284,-0.187531655873748)) ;
#11282=DIRECTION('ref_axis',(0.707106781186548,0.707106781186547,-3.72781918908455E-15)) ;
#11283=DIRECTION('center_axis',(0.376865806842071,-0.90983454207281,0.17370454710351)) ;
#11284=DIRECTION('ref_axis',(0.926267868185696,0.370179664617617,-0.0706742687992895)) ;
#11285=DIRECTION('',(-0.376865806842071,0.90983454207281,-0.17370454710351)) ;
#11286=DIRECTION('center_axis',(4.04047702883407E-15,0.982258559670136,
-0.187531655873747)) ;
#11287=DIRECTION('ref_axis',(1.,-3.98491016764209E-15,7.71272935672663E-16)) ;
#11288=DIRECTION('center_axis',(-0.376865806842073,-0.909834542072809,0.173704547103508)) ;
#11289=DIRECTION('ref_axis',(0.926267868185696,-0.370179664617619,0.0706742687992894)) ;
#11290=DIRECTION('',(0.376865806842073,0.909834542072809,-0.173704547103508)) ;
#11291=DIRECTION('center_axis',(0.694561688421286,0.694561688421282,-0.187531655873747)) ;
#11292=DIRECTION('ref_axis',(0.707106781186545,-0.70710678118655,-2.15313694541952E-15)) ;
#11293=DIRECTION('center_axis',(-0.909834542072809,-0.376865806842072,0.17370454710351)) ;
#11294=DIRECTION('ref_axis',(0.414971211111279,-0.826287510096955,0.380851473157994)) ;
#11295=DIRECTION('',(0.909834542072809,0.376865806842072,-0.17370454710351)) ;
#11296=DIRECTION('center_axis',(0.982258559670136,0.,-0.187531655873751)) ;
#11297=DIRECTION('ref_axis',(-1.261352613548E-15,-1.,-6.42727446393887E-15)) ;
#11298=DIRECTION('center_axis',(0.982258559670136,0.,-0.187531655873751)) ;
#11299=DIRECTION('ref_axis',(-1.261352613548E-15,-1.,-6.42727446393887E-15)) ;
#11300=DIRECTION('center_axis',(-0.90983454207281,0.376865806842072,0.173704547103509)) ;
#11301=DIRECTION('ref_axis',(0.414971211111278,0.826287510096956,0.38085147315799)) ;
#11302=DIRECTION('',(0.90983454207281,-0.376865806842072,-0.173704547103509)) ;
#11303=DIRECTION('center_axis',(0.694561688421279,-0.69456168842129,-0.187531655873747)) ;
#11304=DIRECTION('ref_axis',(0.707106781186553,0.707106781186542,-4.4990921247572E-16)) ;
#11305=DIRECTION('center_axis',(0.694561688421279,-0.69456168842129,-0.187531655873747)) ;
#11306=DIRECTION('ref_axis',(0.707106781186553,0.707106781186542,-4.4990921247572E-16)) ;
#11307=DIRECTION('center_axis',(0.694561688421279,-0.69456168842129,-0.187531655873747)) ;
#11308=DIRECTION('ref_axis',(0.707106781186553,0.707106781186542,-4.4990921247572E-16)) ;
#11309=DIRECTION('center_axis',(-0.376865806842072,0.909834542072809,0.173704547103509)) ;
#11310=DIRECTION('ref_axis',(0.926267868185696,0.370179664617618,0.0706742687992892)) ;
#11311=DIRECTION('',(0.376865806842072,-0.909834542072809,-0.173704547103509)) ;
#11312=DIRECTION('center_axis',(0.,-0.982258559670136,-0.187531655873747)) ;
#11313=DIRECTION('ref_axis',(1.,0.,-8.03409307992359E-18)) ;
#11314=DIRECTION('center_axis',(0.,-0.982258559670136,-0.187531655873747)) ;
#11315=DIRECTION('ref_axis',(1.,0.,-8.03409307992359E-18)) ;
#11316=DIRECTION('center_axis',(0.376865806842073,0.909834542072809,0.173704547103509)) ;
#11317=DIRECTION('ref_axis',(0.926267868185696,-0.370179664617619,-0.0706742687992895)) ;
#11318=DIRECTION('',(-0.376865806842073,-0.909834542072809,-0.173704547103509)) ;
#11319=DIRECTION('center_axis',(-0.69456168842128,-0.694561688421288,-0.187531655873749)) ;
#11320=DIRECTION('ref_axis',(0.707106781186551,-0.707106781186544,6.71650181481614E-15)) ;
#11321=DIRECTION('center_axis',(-0.69456168842128,-0.694561688421288,-0.187531655873749)) ;
#11322=DIRECTION('ref_axis',(0.707106781186551,-0.707106781186544,6.71650181481614E-15)) ;
#11323=DIRECTION('center_axis',(-0.69456168842128,-0.694561688421288,-0.187531655873749)) ;
#11324=DIRECTION('ref_axis',(0.707106781186551,-0.707106781186544,6.71650181481614E-15)) ;
#11325=DIRECTION('center_axis',(0.90983454207281,0.37686580684207,0.173704547103509)) ;
#11326=DIRECTION('ref_axis',(0.414971211111277,-0.826287510096957,-0.380851473157992)) ;
#11327=DIRECTION('',(-0.90983454207281,-0.37686580684207,-0.173704547103509)) ;
#11328=DIRECTION('center_axis',(-0.982258559670136,0.,-0.187531655873751)) ;
#11329=DIRECTION('ref_axis',(-2.45843248245662E-15,-1.,1.2726003438599E-14)) ;
#11330=DIRECTION('center_axis',(-0.982258559670136,0.,-0.187531655873751)) ;
#11331=DIRECTION('ref_axis',(-2.45843248245662E-15,-1.,1.2726003438599E-14)) ;
#11332=DIRECTION('center_axis',(0.909834542072809,-0.376865806842073,0.17370454710351)) ;
#11333=DIRECTION('ref_axis',(0.41497121111128,0.826287510096955,-0.380851473157992)) ;
#11334=DIRECTION('',(-0.909834542072809,0.376865806842073,-0.17370454710351)) ;
#11335=DIRECTION('center_axis',(-0.694561688421284,0.694561688421284,-0.187531655873747)) ;
#11336=DIRECTION('ref_axis',(0.707106781186547,0.707106781186548,2.73159164717402E-15)) ;
#11337=DIRECTION('center_axis',(0.376865806842071,-0.90983454207281,0.173704547103509)) ;
#11338=DIRECTION('ref_axis',(0.926267868185696,0.370179664617617,-0.070674268799289)) ;
#11339=DIRECTION('',(-0.376865806842071,0.90983454207281,-0.173704547103509)) ;
#11340=DIRECTION('center_axis',(6.53814775625694E-15,0.982258559670136,
-0.187531655873747)) ;
#11341=DIRECTION('ref_axis',(1.,-6.42727446393886E-15,1.22118214814838E-15)) ;
#11342=DIRECTION('center_axis',(-0.376865806842073,-0.909834542072809,0.17370454710351)) ;
#11343=DIRECTION('ref_axis',(0.926267868185696,-0.370179664617618,0.0706742687992898)) ;
#11344=DIRECTION('',(0.376865806842073,0.909834542072809,-0.17370454710351)) ;
#11345=DIRECTION('center_axis',(0.694561688421283,0.694561688421285,-0.18753165587375)) ;
#11346=DIRECTION('ref_axis',(0.707106781186548,-0.707106781186547,-7.26282014425093E-15)) ;
#11347=DIRECTION('center_axis',(-0.90983454207281,-0.376865806842071,0.173704547103508)) ;
#11348=DIRECTION('ref_axis',(0.414971211111277,-0.826287510096957,0.38085147315799)) ;
#11349=DIRECTION('',(0.90983454207281,0.376865806842071,-0.173704547103508)) ;
#11350=DIRECTION('center_axis',(0.982258559670137,-8.08095405766815E-15,
-0.187531655873742)) ;
#11351=DIRECTION('ref_axis',(-6.29069488158015E-15,-1.,9.89800267446583E-15)) ;
#11352=DIRECTION('center_axis',(0.982258559670137,-8.08095405766815E-15,
-0.187531655873742)) ;
#11353=DIRECTION('ref_axis',(-6.29069488158015E-15,-1.,9.89800267446583E-15)) ;
#11354=DIRECTION('center_axis',(-0.909834542072809,0.376865806842072,0.17370454710351)) ;
#11355=DIRECTION('ref_axis',(0.414971211111279,0.826287510096955,0.380851473157992)) ;
#11356=DIRECTION('',(0.909834542072809,-0.376865806842072,-0.17370454710351)) ;
#11357=DIRECTION('center_axis',(0.694561688421279,-0.694561688421289,-0.187531655873747)) ;
#11358=DIRECTION('ref_axis',(0.707106781186552,0.707106781186543,-3.3743190935679E-15)) ;
#11359=DIRECTION('center_axis',(0.694561688421279,-0.694561688421289,-0.187531655873747)) ;
#11360=DIRECTION('ref_axis',(0.707106781186552,0.707106781186543,-3.3743190935679E-15)) ;
#11361=DIRECTION('center_axis',(0.694561688421279,-0.694561688421289,-0.187531655873747)) ;
#11362=DIRECTION('ref_axis',(0.707106781186552,0.707106781186543,-3.3743190935679E-15)) ;
#11363=DIRECTION('center_axis',(-0.376865806842072,0.909834542072809,0.173704547103509)) ;
#11364=DIRECTION('ref_axis',(0.926267868185696,0.370179664617618,0.0706742687992893)) ;
#11365=DIRECTION('',(0.376865806842072,-0.909834542072809,-0.173704547103509)) ;
#11366=DIRECTION('center_axis',(-1.5428063014112E-15,-0.982258559670136,
-0.187531655873747)) ;
#11367=DIRECTION('ref_axis',(1.,-1.54254587134533E-15,-3.1332963011702E-16)) ;
#11368=DIRECTION('center_axis',(-1.5428063014112E-15,-0.982258559670136,
-0.187531655873747)) ;
#11369=DIRECTION('ref_axis',(1.,-1.54254587134533E-15,-3.1332963011702E-16)) ;
#11370=DIRECTION('center_axis',(0.376865806842073,0.909834542072809,0.17370454710351)) ;
#11371=DIRECTION('ref_axis',(0.926267868185696,-0.370179664617619,-0.0706742687992899)) ;
#11372=DIRECTION('',(-0.376865806842073,-0.909834542072809,-0.17370454710351)) ;
#11373=DIRECTION('center_axis',(-0.694561688421283,-0.694561688421286,-0.187531655873747)) ;
#11374=DIRECTION('ref_axis',(0.707106781186549,-0.707106781186546,-5.62386515594652E-16)) ;
#11375=DIRECTION('center_axis',(-0.694561688421283,-0.694561688421286,-0.187531655873747)) ;
#11376=DIRECTION('ref_axis',(0.707106781186549,-0.707106781186546,-5.62386515594652E-16)) ;
#11377=DIRECTION('center_axis',(-0.694561688421283,-0.694561688421286,-0.187531655873747)) ;
#11378=DIRECTION('ref_axis',(0.707106781186549,-0.707106781186546,-5.62386515594652E-16)) ;
#11379=DIRECTION('center_axis',(0.90983454207281,0.376865806842072,0.173704547103509)) ;
#11380=DIRECTION('ref_axis',(0.414971211111278,-0.826287510096956,-0.380851473157991)) ;
#11381=DIRECTION('',(-0.90983454207281,-0.376865806842072,-0.173704547103509)) ;
#11382=DIRECTION('center_axis',(-0.982258559670137,0.,-0.187531655873742)) ;
#11383=DIRECTION('ref_axis',(2.10493238693998E-15,-1.,-1.10549120779749E-14)) ;
#11384=DIRECTION('center_axis',(-0.982258559670137,0.,-0.187531655873742)) ;
#11385=DIRECTION('ref_axis',(2.10493238693998E-15,-1.,-1.10549120779749E-14)) ;
#11386=DIRECTION('center_axis',(0.90983454207281,-0.376865806842072,0.173704547103508)) ;
#11387=DIRECTION('ref_axis',(0.414971211111278,0.826287510096957,-0.380851473157989)) ;
#11388=DIRECTION('',(-0.90983454207281,0.376865806842072,-0.173704547103508)) ;
#11389=DIRECTION('center_axis',(-0.694561688421283,0.694561688421285,-0.187531655873748)) ;
#11390=DIRECTION('ref_axis',(0.707106781186549,0.707106781186546,-3.9849101676421E-15)) ;
#11391=DIRECTION('center_axis',(0.376865806842071,-0.90983454207281,0.173704547103509)) ;
#11392=DIRECTION('ref_axis',(0.926267868185696,0.370179664617617,-0.0706742687992893)) ;
#11393=DIRECTION('',(-0.376865806842071,0.90983454207281,-0.173704547103509)) ;
#11394=DIRECTION('center_axis',(4.04047702883407E-15,0.982258559670136,
-0.187531655873749)) ;
#11395=DIRECTION('ref_axis',(1.,-3.98491016764209E-15,7.6323884259274E-16)) ;
#11396=DIRECTION('center_axis',(-0.376865806842073,-0.909834542072809,0.173704547103509)) ;
#11397=DIRECTION('ref_axis',(0.926267868185696,-0.370179664617619,0.0706742687992897)) ;
#11398=DIRECTION('',(0.376865806842073,0.909834542072809,-0.173704547103509)) ;
#11399=DIRECTION('center_axis',(0.694561688421284,0.694561688421285,-0.187531655873748)) ;
#11400=DIRECTION('ref_axis',(0.707106781186548,-0.707106781186547,-2.8601371364528E-15)) ;
#11401=DIRECTION('center_axis',(-0.90983454207281,-0.376865806842072,0.17370454710351)) ;
#11402=DIRECTION('ref_axis',(0.414971211111278,-0.826287510096955,0.380851473157992)) ;
#11403=DIRECTION('',(0.909834542072809,0.376865806842072,-0.17370454710351)) ;
#11404=DIRECTION('center_axis',(0.982258559670137,0.,-0.187531655873743)) ;
#11405=DIRECTION('ref_axis',(1.94425052534151E-15,-1.,1.05407301208597E-14)) ;
#11406=DIRECTION('center_axis',(0.982258559670137,0.,-0.187531655873743)) ;
#11407=DIRECTION('ref_axis',(1.94425052534151E-15,-1.,1.05407301208597E-14)) ;
#11408=DIRECTION('center_axis',(-0.909834542072809,0.376865806842072,0.173704547103509)) ;
#11409=DIRECTION('ref_axis',(0.414971211111278,0.826287510096956,0.38085147315799)) ;
#11410=DIRECTION('',(0.909834542072809,-0.376865806842072,-0.173704547103509)) ;
#11411=DIRECTION('center_axis',(0.69456168842128,-0.694561688421288,-0.187531655873748)) ;
#11412=DIRECTION('ref_axis',(0.707106781186552,0.707106781186543,1.83177322222257E-15)) ;
#11413=DIRECTION('center_axis',(0.69456168842128,-0.694561688421288,-0.187531655873748)) ;
#11414=DIRECTION('ref_axis',(0.707106781186552,0.707106781186543,1.83177322222257E-15)) ;
#11415=DIRECTION('center_axis',(0.69456168842128,-0.694561688421288,-0.187531655873748)) ;
#11416=DIRECTION('ref_axis',(0.707106781186552,0.707106781186543,1.83177322222257E-15)) ;
#11417=DIRECTION('center_axis',(-0.376865806842072,0.909834542072809,0.173704547103509)) ;
#11418=DIRECTION('ref_axis',(0.926267868185696,0.370179664617618,0.0706742687992893)) ;
#11419=DIRECTION('',(0.376865806842072,-0.909834542072809,-0.173704547103509)) ;
#11420=DIRECTION('center_axis',(-7.71403150705611E-16,-0.982258559670136,
-0.187531655873747)) ;
#11421=DIRECTION('ref_axis',(1.,-8.35545680312053E-16,-1.76750047758319E-16)) ;
#11422=DIRECTION('center_axis',(-7.71403150705611E-16,-0.982258559670136,
-0.187531655873747)) ;
#11423=DIRECTION('ref_axis',(1.,-8.35545680312053E-16,-1.76750047758319E-16)) ;
#11424=DIRECTION('center_axis',(0.376865806842073,0.909834542072809,0.173704547103509)) ;
#11425=DIRECTION('ref_axis',(0.926267868185696,-0.370179664617618,-0.0706742687992894)) ;
#11426=DIRECTION('',(-0.376865806842073,-0.909834542072809,-0.173704547103509)) ;
#11427=DIRECTION('center_axis',(-0.694561688421285,-0.694561688421283,-0.187531655873748)) ;
#11428=DIRECTION('ref_axis',(0.707106781186546,-0.707106781186549,3.31004634892852E-15)) ;
#11429=DIRECTION('center_axis',(-0.694561688421285,-0.694561688421283,-0.187531655873748)) ;
#11430=DIRECTION('ref_axis',(0.707106781186546,-0.707106781186549,3.31004634892852E-15)) ;
#11431=DIRECTION('center_axis',(-0.694561688421285,-0.694561688421283,-0.187531655873748)) ;
#11432=DIRECTION('ref_axis',(0.707106781186546,-0.707106781186549,3.31004634892852E-15)) ;
#11433=DIRECTION('center_axis',(0.909834542072809,0.376865806842072,0.173704547103509)) ;
#11434=DIRECTION('ref_axis',(0.414971211111279,-0.826287510096956,-0.380851473157991)) ;
#11435=DIRECTION('',(-0.909834542072809,-0.376865806842072,-0.173704547103509)) ;
#11436=DIRECTION('center_axis',(-0.982258559670137,0.,-0.187531655873743)) ;
#11437=DIRECTION('ref_axis',(1.82373912914265E-15,-1.,-9.70518444054769E-15)) ;
#11438=DIRECTION('center_axis',(-0.982258559670137,0.,-0.187531655873743)) ;
#11439=DIRECTION('ref_axis',(1.82373912914265E-15,-1.,-9.70518444054769E-15)) ;
#11440=DIRECTION('center_axis',(0.90983454207281,-0.376865806842072,0.173704547103509)) ;
#11441=DIRECTION('ref_axis',(0.414971211111278,0.826287510096956,-0.380851473157991)) ;
#11442=DIRECTION('',(-0.90983454207281,0.376865806842072,-0.173704547103509)) ;
#11443=DIRECTION('center_axis',(-0.694561688421285,0.694561688421283,-0.18753165587375)) ;
#11444=DIRECTION('ref_axis',(0.707106781186547,0.707106781186548,-6.10591074074193E-15)) ;
#11445=DIRECTION('center_axis',(0.376865806842071,-0.90983454207281,0.173704547103509)) ;
#11446=DIRECTION('ref_axis',(0.926267868185696,0.370179664617617,-0.0706742687992893)) ;
#11447=DIRECTION('',(-0.376865806842071,0.90983454207281,-0.173704547103509)) ;
#11448=DIRECTION('center_axis',(4.81188017953967E-15,0.982258559670136,
-0.187531655873747)) ;
#11449=DIRECTION('ref_axis',(1.,-4.75618310331476E-15,9.15886611111287E-16)) ;
#11450=DIRECTION('center_axis',(-0.376865806842072,-0.90983454207281,0.173704547103509)) ;
#11451=DIRECTION('ref_axis',(0.926267868185696,-0.370179664617617,0.0706742687992892)) ;
#11452=DIRECTION('',(0.376865806842072,0.90983454207281,-0.173704547103509)) ;
#11453=DIRECTION('center_axis',(0.694561688421281,0.694561688421287,-0.187531655873748)) ;
#11454=DIRECTION('ref_axis',(0.70710678118655,-0.707106781186545,-3.90456923684287E-15)) ;
#11455=DIRECTION('center_axis',(-0.90983454207281,-0.376865806842072,0.173704547103509)) ;
#11456=DIRECTION('ref_axis',(0.414971211111278,-0.826287510096956,0.380851473157991)) ;
#11457=DIRECTION('',(0.909834542072809,0.376865806842072,-0.173704547103509)) ;
#11458=DIRECTION('center_axis',(0.982258559670137,-8.85235720837373E-15,
-0.187531655873743)) ;
#11459=DIRECTION('ref_axis',(-6.81291093177518E-15,-1.,1.11834575672536E-14)) ;
#11460=DIRECTION('center_axis',(0.982258559670137,-8.85235720837373E-15,
-0.187531655873743)) ;
#11461=DIRECTION('ref_axis',(-6.81291093177518E-15,-1.,1.11834575672536E-14)) ;
#11462=DIRECTION('center_axis',(-0.909834542072809,0.376865806842072,0.173704547103509)) ;
#11463=DIRECTION('ref_axis',(0.414971211111278,0.826287510096956,0.38085147315799)) ;
#11464=DIRECTION('',(0.909834542072809,-0.376865806842072,-0.173704547103509)) ;
#11465=DIRECTION('center_axis',(0.694561688421281,-0.694561688421288,-0.187531655873748)) ;
#11466=DIRECTION('ref_axis',(0.707106781186551,0.707106781186544,2.18527331773921E-15)) ;
#11467=DIRECTION('center_axis',(0.694561688421281,-0.694561688421288,-0.187531655873748)) ;
#11468=DIRECTION('ref_axis',(0.707106781186551,0.707106781186544,2.18527331773921E-15)) ;
#11469=DIRECTION('center_axis',(0.694561688421281,-0.694561688421288,-0.187531655873748)) ;
#11470=DIRECTION('ref_axis',(0.707106781186551,0.707106781186544,2.18527331773921E-15)) ;
#11471=DIRECTION('center_axis',(-0.376865806842073,0.909834542072809,0.173704547103509)) ;
#11472=DIRECTION('ref_axis',(0.926267868185696,0.370179664617618,0.0706742687992896)) ;
#11473=DIRECTION('',(0.376865806842073,-0.909834542072809,-0.173704547103509)) ;
#11474=DIRECTION('center_axis',(0.376865806842073,-0.909834542072809,-0.173704547103509)) ;
#11475=DIRECTION('ref_axis',(0.926267868185696,0.370179664617618,0.0706742687992896)) ;
#11476=DIRECTION('center_axis',(0.376865806842073,-0.909834542072809,-0.173704547103509)) ;
#11477=DIRECTION('ref_axis',(-0.926267868185696,-0.370179664617618,-0.0706742687992896)) ;
#13783=CARTESIAN_POINT('',(0.,0.,0.)) ;
#13784=CARTESIAN_POINT('Origin',(-1.32322330470336,0.523223304703363,1.87625)) ;
#13785=CARTESIAN_POINT('',(-1.31990818206448,0.52653842734225,1.85169353600825)) ;
#13786=CARTESIAN_POINT('',(-1.32653842734225,0.519908182064476,1.90080646399175)) ;
#13787=CARTESIAN_POINT('Origin',(-1.32322330470336,0.523223304703363,1.87625)) ;
#13788=CARTESIAN_POINT('Origin',(-1.32322330470336,0.523223304703363,1.87625)) ;
#13789=CARTESIAN_POINT('Origin',(-1.5,0.45,1.8425)) ;
#13790=CARTESIAN_POINT('',(-1.49531170860316,0.45,1.81794353600825)) ;
#13791=CARTESIAN_POINT('',(-1.50468829139684,0.45,1.86705646399175)) ;
#13792=CARTESIAN_POINT('Origin',(-1.5,0.45,1.8425)) ;
#13793=CARTESIAN_POINT('',(-1.51037428027778,0.429342812247576,1.85202128682895)) ;
#13794=CARTESIAN_POINT('Origin',(-1.5,0.45,1.8425)) ;
#13795=CARTESIAN_POINT('Origin',(-1.5,0.45,1.8425)) ;
#13796=CARTESIAN_POINT('Origin',(-1.67677669529664,0.523223304703363,1.80875)) ;
#13797=CARTESIAN_POINT('',(-1.67346157265775,0.519908182064476,1.78419353600825)) ;
#13798=CARTESIAN_POINT('',(-1.68715097557442,0.502566116950939,1.81827128682895)) ;
#13799=CARTESIAN_POINT('Origin',(-1.67677669529664,0.523223304703363,1.80875)) ;
#13800=CARTESIAN_POINT('',(-1.68009181793552,0.52653842734225,1.83330646399175)) ;
#13801=CARTESIAN_POINT('Origin',(-1.67677669529664,0.523223304703363,1.80875)) ;
#13802=CARTESIAN_POINT('',(-1.69993339200128,0.513968813087923,1.81051685671998)) ;
#13803=CARTESIAN_POINT('Origin',(-1.67677669529664,0.523223304703363,1.80875)) ;
#13804=CARTESIAN_POINT('Origin',(-1.67677669529664,0.523223304703363,1.80875)) ;
#13805=CARTESIAN_POINT('Origin',(-1.75,0.7,1.775)) ;
#13806=CARTESIAN_POINT('',(-1.75,0.695311708603157,1.75044353600825)) ;
#13807=CARTESIAN_POINT('',(-1.77315669670464,0.69074550838456,1.77676685671998)) ;
#13808=CARTESIAN_POINT('Origin',(-1.75,0.7,1.775)) ;
#13809=CARTESIAN_POINT('',(-1.75,0.704688291396844,1.79955646399175)) ;
#13810=CARTESIAN_POINT('Origin',(-1.75,0.7,1.775)) ;
#13811=CARTESIAN_POINT('',(-1.77315669670464,0.709254491615441,1.77323314328002)) ;
#13812=CARTESIAN_POINT('Origin',(-1.75,0.7,1.775)) ;
#13813=CARTESIAN_POINT('Origin',(-1.75,0.7,1.775)) ;
#13814=CARTESIAN_POINT('Origin',(-1.67677669529664,0.876776695296637,1.74125)) ;
#13815=CARTESIAN_POINT('',(-1.68009181793552,0.873461572657751,1.71669353600825)) ;
#13816=CARTESIAN_POINT('',(-1.69993339200128,0.886031186912078,1.73948314328002)) ;
#13817=CARTESIAN_POINT('Origin',(-1.67677669529664,0.876776695296637,1.74125)) ;
#13818=CARTESIAN_POINT('',(-1.67346157265775,0.880091817935524,1.76580646399175)) ;
#13819=CARTESIAN_POINT('Origin',(-1.67677669529664,0.876776695296637,1.74125)) ;
#13820=CARTESIAN_POINT('',(-1.68715097557442,0.897433883049061,1.73172871317105)) ;
#13821=CARTESIAN_POINT('Origin',(-1.67677669529664,0.876776695296637,1.74125)) ;
#13822=CARTESIAN_POINT('Origin',(-1.67677669529664,0.876776695296637,1.74125)) ;
#13823=CARTESIAN_POINT('Origin',(-1.5,0.95,1.7075)) ;
#13824=CARTESIAN_POINT('',(-1.50468829139684,0.95,1.68294353600825)) ;
#13825=CARTESIAN_POINT('',(-1.51037428027778,0.970657187752424,1.69797871317105)) ;
#13826=CARTESIAN_POINT('Origin',(-1.5,0.95,1.7075)) ;
#13827=CARTESIAN_POINT('',(-1.49531170860316,0.95,1.73205646399175)) ;
#13828=CARTESIAN_POINT('Origin',(-1.5,0.95,1.7075)) ;
#13829=CARTESIAN_POINT('Origin',(-1.5,0.95,1.7075)) ;
#13830=CARTESIAN_POINT('Origin',(-1.32322330470336,0.876776695296637,1.67375)) ;
#13831=CARTESIAN_POINT('',(-1.32653842734225,0.880091817935524,1.64919353600825)) ;
#13832=CARTESIAN_POINT('',(-1.31990818206448,0.87346157265775,1.69830646399175)) ;
#13833=CARTESIAN_POINT('Origin',(-1.32322330470336,0.876776695296637,1.67375)) ;
#13834=CARTESIAN_POINT('Origin',(-1.32322330470336,0.876776695296637,1.67375)) ;
#13835=CARTESIAN_POINT('Origin',(-1.25,0.7,1.64)) ;
#13836=CARTESIAN_POINT('',(-1.25,0.704688291396843,1.61544353600825)) ;
#13837=CARTESIAN_POINT('',(-1.25,0.695311708603156,1.66455646399175)) ;
#13838=CARTESIAN_POINT('Origin',(-1.25,0.7,1.64)) ;
#13839=CARTESIAN_POINT('Origin',(-1.25,0.7,1.64)) ;
#13840=CARTESIAN_POINT('Origin',(-1.32322330470336,0.523223304703363,1.60625)) ;
#13841=CARTESIAN_POINT('',(-1.31990818206448,0.52653842734225,1.58169353600825)) ;
#13842=CARTESIAN_POINT('',(-1.32653842734225,0.519908182064476,1.63080646399175)) ;
#13843=CARTESIAN_POINT('Origin',(-1.32322330470336,0.523223304703363,1.60625)) ;
#13844=CARTESIAN_POINT('Origin',(-1.32322330470336,0.523223304703363,1.60625)) ;
#13845=CARTESIAN_POINT('Origin',(-1.5,0.45,1.5725)) ;
#13846=CARTESIAN_POINT('',(-1.49531170860316,0.45,1.54794353600825)) ;
#13847=CARTESIAN_POINT('',(-1.50468829139684,0.45,1.59705646399175)) ;
#13848=CARTESIAN_POINT('Origin',(-1.5,0.45,1.5725)) ;
#13849=CARTESIAN_POINT('',(-1.51037428027778,0.429342812247576,1.58202128682895)) ;
#13850=CARTESIAN_POINT('Origin',(-1.5,0.45,1.5725)) ;
#13851=CARTESIAN_POINT('Origin',(-1.5,0.45,1.5725)) ;
#13852=CARTESIAN_POINT('Origin',(-1.67677669529664,0.523223304703363,1.53875)) ;
#13853=CARTESIAN_POINT('',(-1.67346157265775,0.519908182064476,1.51419353600825)) ;
#13854=CARTESIAN_POINT('',(-1.68715097557442,0.502566116950939,1.54827128682895)) ;
#13855=CARTESIAN_POINT('Origin',(-1.67677669529664,0.523223304703363,1.53875)) ;
#13856=CARTESIAN_POINT('',(-1.68009181793552,0.52653842734225,1.56330646399175)) ;
#13857=CARTESIAN_POINT('Origin',(-1.67677669529664,0.523223304703363,1.53875)) ;
#13858=CARTESIAN_POINT('',(-1.69993339200128,0.513968813087923,1.54051685671998)) ;
#13859=CARTESIAN_POINT('Origin',(-1.67677669529664,0.523223304703363,1.53875)) ;
#13860=CARTESIAN_POINT('Origin',(-1.67677669529664,0.523223304703363,1.53875)) ;
#13861=CARTESIAN_POINT('Origin',(-1.75,0.7,1.505)) ;
#13862=CARTESIAN_POINT('',(-1.75,0.695311708603156,1.48044353600825)) ;
#13863=CARTESIAN_POINT('',(-1.77315669670464,0.69074550838456,1.50676685671998)) ;
#13864=CARTESIAN_POINT('Origin',(-1.75,0.7,1.505)) ;
#13865=CARTESIAN_POINT('',(-1.75,0.704688291396844,1.52955646399175)) ;
#13866=CARTESIAN_POINT('Origin',(-1.75,0.7,1.505)) ;
#13867=CARTESIAN_POINT('',(-1.77315669670464,0.709254491615441,1.50323314328002)) ;
#13868=CARTESIAN_POINT('Origin',(-1.75,0.7,1.505)) ;
#13869=CARTESIAN_POINT('Origin',(-1.75,0.7,1.505)) ;
#13870=CARTESIAN_POINT('Origin',(-1.67677669529664,0.876776695296637,1.47125)) ;
#13871=CARTESIAN_POINT('',(-1.68009181793552,0.87346157265775,1.44669353600825)) ;
#13872=CARTESIAN_POINT('',(-1.69993339200128,0.886031186912078,1.46948314328002)) ;
#13873=CARTESIAN_POINT('Origin',(-1.67677669529664,0.876776695296637,1.47125)) ;
#13874=CARTESIAN_POINT('',(-1.67346157265775,0.880091817935524,1.49580646399175)) ;
#13875=CARTESIAN_POINT('Origin',(-1.67677669529664,0.876776695296637,1.47125)) ;
#13876=CARTESIAN_POINT('',(-1.68715097557442,0.897433883049061,1.46172871317105)) ;
#13877=CARTESIAN_POINT('Origin',(-1.67677669529664,0.876776695296637,1.47125)) ;
#13878=CARTESIAN_POINT('Origin',(-1.67677669529664,0.876776695296637,1.47125)) ;
#13879=CARTESIAN_POINT('Origin',(-1.5,0.95,1.4375)) ;
#13880=CARTESIAN_POINT('',(-1.50468829139684,0.95,1.41294353600825)) ;
#13881=CARTESIAN_POINT('',(-1.51037428027778,0.970657187752424,1.42797871317105)) ;
#13882=CARTESIAN_POINT('Origin',(-1.5,0.95,1.4375)) ;
#13883=CARTESIAN_POINT('',(-1.49531170860316,0.95,1.46205646399175)) ;
#13884=CARTESIAN_POINT('Origin',(-1.5,0.95,1.4375)) ;
#13885=CARTESIAN_POINT('Origin',(-1.5,0.95,1.4375)) ;
#13886=CARTESIAN_POINT('Origin',(-1.32322330470336,0.876776695296637,1.40375)) ;
#13887=CARTESIAN_POINT('',(-1.32653842734225,0.880091817935524,1.37919353600825)) ;
#13888=CARTESIAN_POINT('',(-1.31990818206448,0.87346157265775,1.42830646399175)) ;
#13889=CARTESIAN_POINT('Origin',(-1.32322330470336,0.876776695296637,1.40375)) ;
#13890=CARTESIAN_POINT('Origin',(-1.32322330470336,0.876776695296637,1.40375)) ;
#13891=CARTESIAN_POINT('Origin',(-1.25,0.7,1.37)) ;
#13892=CARTESIAN_POINT('',(-1.25,0.704688291396844,1.34544353600825)) ;
#13893=CARTESIAN_POINT('',(-1.25,0.695311708603156,1.39455646399175)) ;
#13894=CARTESIAN_POINT('Origin',(-1.25,0.7,1.37)) ;
#13895=CARTESIAN_POINT('Origin',(-1.25,0.7,1.37)) ;
#13896=CARTESIAN_POINT('Origin',(-1.32322330470336,0.523223304703363,1.33625)) ;
#13897=CARTESIAN_POINT('',(-1.31990818206448,0.52653842734225,1.31169353600825)) ;
#13898=CARTESIAN_POINT('',(-1.32653842734225,0.519908182064476,1.36080646399175)) ;
#13899=CARTESIAN_POINT('Origin',(-1.32322330470336,0.523223304703363,1.33625)) ;
#13900=CARTESIAN_POINT('Origin',(-1.32322330470336,0.523223304703363,1.33625)) ;
#13901=CARTESIAN_POINT('Origin',(-1.5,0.45,1.3025)) ;
#13902=CARTESIAN_POINT('',(-1.49531170860316,0.45,1.27794353600825)) ;
#13903=CARTESIAN_POINT('',(-1.50468829139684,0.45,1.32705646399175)) ;
#13904=CARTESIAN_POINT('Origin',(-1.5,0.45,1.3025)) ;
#13905=CARTESIAN_POINT('',(-1.51037428027778,0.429342812247576,1.31202128682895)) ;
#13906=CARTESIAN_POINT('Origin',(-1.5,0.45,1.3025)) ;
#13907=CARTESIAN_POINT('Origin',(-1.5,0.45,1.3025)) ;
#13908=CARTESIAN_POINT('Origin',(-1.67677669529664,0.523223304703363,1.26875)) ;
#13909=CARTESIAN_POINT('',(-1.67346157265775,0.519908182064476,1.24419353600825)) ;
#13910=CARTESIAN_POINT('',(-1.68715097557442,0.502566116950939,1.27827128682895)) ;
#13911=CARTESIAN_POINT('Origin',(-1.67677669529664,0.523223304703363,1.26875)) ;
#13912=CARTESIAN_POINT('',(-1.68009181793552,0.52653842734225,1.29330646399175)) ;
#13913=CARTESIAN_POINT('Origin',(-1.67677669529664,0.523223304703363,1.26875)) ;
#13914=CARTESIAN_POINT('',(-1.69993339200128,0.513968813087923,1.27051685671998)) ;
#13915=CARTESIAN_POINT('Origin',(-1.67677669529664,0.523223304703363,1.26875)) ;
#13916=CARTESIAN_POINT('Origin',(-1.67677669529664,0.523223304703363,1.26875)) ;
#13917=CARTESIAN_POINT('Origin',(-1.75,0.7,1.235)) ;
#13918=CARTESIAN_POINT('',(-1.75,0.695311708603157,1.21044353600825)) ;
#13919=CARTESIAN_POINT('',(-1.77315669670464,0.69074550838456,1.23676685671998)) ;
#13920=CARTESIAN_POINT('Origin',(-1.75,0.7,1.235)) ;
#13921=CARTESIAN_POINT('',(-1.75,0.704688291396844,1.25955646399175)) ;
#13922=CARTESIAN_POINT('Origin',(-1.75,0.7,1.235)) ;
#13923=CARTESIAN_POINT('',(-1.77315669670464,0.70925449161544,1.23323314328002)) ;
#13924=CARTESIAN_POINT('Origin',(-1.75,0.7,1.235)) ;
#13925=CARTESIAN_POINT('Origin',(-1.75,0.7,1.235)) ;
#13926=CARTESIAN_POINT('Origin',(-1.67677669529664,0.876776695296637,1.20125)) ;
#13927=CARTESIAN_POINT('',(-1.68009181793552,0.87346157265775,1.17669353600825)) ;
#13928=CARTESIAN_POINT('',(-1.69993339200128,0.886031186912078,1.19948314328002)) ;
#13929=CARTESIAN_POINT('Origin',(-1.67677669529664,0.876776695296637,1.20125)) ;
#13930=CARTESIAN_POINT('',(-1.67346157265775,0.880091817935524,1.22580646399175)) ;
#13931=CARTESIAN_POINT('Origin',(-1.67677669529664,0.876776695296637,1.20125)) ;
#13932=CARTESIAN_POINT('',(-1.68715097557442,0.897433883049061,1.19172871317105)) ;
#13933=CARTESIAN_POINT('Origin',(-1.67677669529664,0.876776695296637,1.20125)) ;
#13934=CARTESIAN_POINT('Origin',(-1.67677669529664,0.876776695296637,1.20125)) ;
#13935=CARTESIAN_POINT('Origin',(-1.5,0.95,1.1675)) ;
#13936=CARTESIAN_POINT('',(-1.50468829139684,0.95,1.14294353600825)) ;
#13937=CARTESIAN_POINT('',(-1.51037428027778,0.970657187752424,1.15797871317105)) ;
#13938=CARTESIAN_POINT('Origin',(-1.5,0.95,1.1675)) ;
#13939=CARTESIAN_POINT('',(-1.49531170860316,0.95,1.19205646399175)) ;
#13940=CARTESIAN_POINT('Origin',(-1.5,0.95,1.1675)) ;
#13941=CARTESIAN_POINT('Origin',(-1.5,0.95,1.1675)) ;
#13942=CARTESIAN_POINT('Origin',(-1.32322330470336,0.876776695296637,1.13375)) ;
#13943=CARTESIAN_POINT('',(-1.32653842734225,0.880091817935524,1.10919353600825)) ;
#13944=CARTESIAN_POINT('',(-1.31990818206448,0.87346157265775,1.15830646399175)) ;
#13945=CARTESIAN_POINT('Origin',(-1.32322330470336,0.876776695296637,1.13375)) ;
#13946=CARTESIAN_POINT('Origin',(-1.32322330470336,0.876776695296637,1.13375)) ;
#13947=CARTESIAN_POINT('Origin',(-1.25,0.7,1.1)) ;
#13948=CARTESIAN_POINT('',(-1.25,0.704688291396844,1.07544353600825)) ;
#13949=CARTESIAN_POINT('',(-1.25,0.695311708603156,1.12455646399175)) ;
#13950=CARTESIAN_POINT('Origin',(-1.25,0.7,1.1)) ;
#13951=CARTESIAN_POINT('Origin',(-1.25,0.7,1.1)) ;
#13952=CARTESIAN_POINT('Origin',(-1.32322330470336,0.523223304703363,1.06625)) ;
#13953=CARTESIAN_POINT('',(-1.31990818206448,0.52653842734225,1.04169353600825)) ;
#13954=CARTESIAN_POINT('',(-1.32653842734225,0.519908182064476,1.09080646399175)) ;
#13955=CARTESIAN_POINT('Origin',(-1.32322330470336,0.523223304703363,1.06625)) ;
#13956=CARTESIAN_POINT('Origin',(-1.32322330470336,0.523223304703363,1.06625)) ;
#13957=CARTESIAN_POINT('Origin',(-1.5,0.45,1.0325)) ;
#13958=CARTESIAN_POINT('',(-1.49531170860316,0.45,1.00794353600825)) ;
#13959=CARTESIAN_POINT('',(-1.50468829139684,0.45,1.05705646399175)) ;
#13960=CARTESIAN_POINT('Origin',(-1.5,0.45,1.0325)) ;
#13961=CARTESIAN_POINT('',(-1.51037428027778,0.429342812247576,1.04202128682895)) ;
#13962=CARTESIAN_POINT('Origin',(-1.5,0.45,1.0325)) ;
#13963=CARTESIAN_POINT('Origin',(-1.5,0.45,1.0325)) ;
#13964=CARTESIAN_POINT('Origin',(-1.67677669529664,0.523223304703363,0.99875)) ;
#13965=CARTESIAN_POINT('',(-1.67346157265775,0.519908182064476,0.974193536008247)) ;
#13966=CARTESIAN_POINT('',(-1.68715097557442,0.502566116950939,1.00827128682895)) ;
#13967=CARTESIAN_POINT('Origin',(-1.67677669529664,0.523223304703363,0.99875)) ;
#13968=CARTESIAN_POINT('',(-1.68009181793552,0.52653842734225,1.02330646399175)) ;
#13969=CARTESIAN_POINT('Origin',(-1.67677669529664,0.523223304703363,0.99875)) ;
#13970=CARTESIAN_POINT('',(-1.69993339200128,0.513968813087922,1.00051685671998)) ;
#13971=CARTESIAN_POINT('Origin',(-1.67677669529664,0.523223304703363,0.99875)) ;
#13972=CARTESIAN_POINT('Origin',(-1.67677669529664,0.523223304703363,0.99875)) ;
#13973=CARTESIAN_POINT('Origin',(-1.75,0.7,0.965)) ;
#13974=CARTESIAN_POINT('',(-1.75,0.695311708603157,0.940443536008247)) ;
#13975=CARTESIAN_POINT('',(-1.77315669670464,0.69074550838456,0.966766856719982)) ;
#13976=CARTESIAN_POINT('Origin',(-1.75,0.7,0.965)) ;
#13977=CARTESIAN_POINT('',(-1.75,0.704688291396844,0.989556463991753)) ;
#13978=CARTESIAN_POINT('Origin',(-1.75,0.7,0.965)) ;
#13979=CARTESIAN_POINT('',(-1.77315669670464,0.709254491615441,0.963233143280018)) ;
#13980=CARTESIAN_POINT('Origin',(-1.75,0.7,0.965)) ;
#13981=CARTESIAN_POINT('Origin',(-1.75,0.7,0.965)) ;
#13982=CARTESIAN_POINT('Origin',(-1.67677669529664,0.876776695296637,0.93125)) ;
#13983=CARTESIAN_POINT('',(-1.68009181793552,0.87346157265775,0.906693536008247)) ;
#13984=CARTESIAN_POINT('',(-1.69993339200128,0.886031186912078,0.929483143280018)) ;
#13985=CARTESIAN_POINT('Origin',(-1.67677669529664,0.876776695296637,0.93125)) ;
#13986=CARTESIAN_POINT('',(-1.67346157265775,0.880091817935524,0.955806463991753)) ;
#13987=CARTESIAN_POINT('Origin',(-1.67677669529664,0.876776695296637,0.93125)) ;
#13988=CARTESIAN_POINT('',(-1.68715097557442,0.897433883049061,0.92172871317105)) ;
#13989=CARTESIAN_POINT('Origin',(-1.67677669529664,0.876776695296637,0.93125)) ;
#13990=CARTESIAN_POINT('Origin',(-1.67677669529664,0.876776695296637,0.93125)) ;
#13991=CARTESIAN_POINT('Origin',(-1.5,0.95,0.8975)) ;
#13992=CARTESIAN_POINT('',(-1.50468829139684,0.95,0.872943536008246)) ;
#13993=CARTESIAN_POINT('',(-1.51037428027778,0.970657187752424,0.88797871317105)) ;
#13994=CARTESIAN_POINT('Origin',(-1.5,0.95,0.8975)) ;
#13995=CARTESIAN_POINT('',(-1.49531170860316,0.950000000000001,0.922056463991753)) ;
#13996=CARTESIAN_POINT('Origin',(-1.5,0.95,0.8975)) ;
#13997=CARTESIAN_POINT('Origin',(-1.5,0.95,0.8975)) ;
#13998=CARTESIAN_POINT('Origin',(-1.32322330470336,0.876776695296637,0.86375)) ;
#13999=CARTESIAN_POINT('',(-1.32653842734225,0.880091817935523,0.839193536008247)) ;
#14000=CARTESIAN_POINT('',(-1.31990818206448,0.87346157265775,0.888306463991753)) ;
#14001=CARTESIAN_POINT('Origin',(-1.32322330470336,0.876776695296637,0.86375)) ;
#14002=CARTESIAN_POINT('Origin',(-1.32322330470336,0.876776695296637,0.86375)) ;
#14003=CARTESIAN_POINT('Origin',(-1.25,0.7,0.83)) ;
#14004=CARTESIAN_POINT('',(-1.25,0.704688291396844,0.805443536008247)) ;
#14005=CARTESIAN_POINT('',(-1.25,0.695311708603156,0.854556463991753)) ;
#14006=CARTESIAN_POINT('Origin',(-1.25,0.7,0.83)) ;
#14007=CARTESIAN_POINT('Origin',(-1.25,0.7,0.83)) ;
#14008=CARTESIAN_POINT('Origin',(-1.32322330470336,0.523223304703363,0.79625)) ;
#14009=CARTESIAN_POINT('',(-1.31990818206448,0.52653842734225,0.771693536008247)) ;
#14010=CARTESIAN_POINT('',(-1.32653842734225,0.519908182064476,0.820806463991753)) ;
#14011=CARTESIAN_POINT('Origin',(-1.32322330470336,0.523223304703363,0.79625)) ;
#14012=CARTESIAN_POINT('Origin',(-1.32322330470336,0.523223304703363,0.79625)) ;
#14013=CARTESIAN_POINT('Origin',(-1.5,0.45,0.7625)) ;
#14014=CARTESIAN_POINT('',(-1.49531170860316,0.45,0.737943536008247)) ;
#14015=CARTESIAN_POINT('',(-1.50468829139684,0.45,0.787056463991754)) ;
#14016=CARTESIAN_POINT('Origin',(-1.5,0.45,0.7625)) ;
#14017=CARTESIAN_POINT('',(-1.51037428027778,0.429342812247576,0.77202128682895)) ;
#14018=CARTESIAN_POINT('Origin',(-1.5,0.45,0.7625)) ;
#14019=CARTESIAN_POINT('Origin',(-1.5,0.45,0.7625)) ;
#14020=CARTESIAN_POINT('Origin',(-1.67677669529664,0.523223304703363,0.72875)) ;
#14021=CARTESIAN_POINT('',(-1.67346157265775,0.519908182064476,0.704193536008247)) ;
#14022=CARTESIAN_POINT('',(-1.68715097557442,0.502566116950939,0.73827128682895)) ;
#14023=CARTESIAN_POINT('Origin',(-1.67677669529664,0.523223304703363,0.72875)) ;
#14024=CARTESIAN_POINT('',(-1.68009181793552,0.52653842734225,0.753306463991753)) ;
#14025=CARTESIAN_POINT('Origin',(-1.67677669529664,0.523223304703363,0.72875)) ;
#14026=CARTESIAN_POINT('',(-1.69993339200128,0.513968813087923,0.730516856719982)) ;
#14027=CARTESIAN_POINT('Origin',(-1.67677669529664,0.523223304703363,0.72875)) ;
#14028=CARTESIAN_POINT('Origin',(-1.67677669529664,0.523223304703363,0.72875)) ;
#14029=CARTESIAN_POINT('Origin',(-1.75,0.7,0.695)) ;
#14030=CARTESIAN_POINT('',(-1.75,0.695311708603156,0.670443536008247)) ;
#14031=CARTESIAN_POINT('',(-1.77315669670464,0.69074550838456,0.696766856719982)) ;
#14032=CARTESIAN_POINT('Origin',(-1.75,0.7,0.695)) ;
#14033=CARTESIAN_POINT('',(-1.75,0.704688291396844,0.719556463991753)) ;
#14034=CARTESIAN_POINT('Origin',(-1.75,0.7,0.695)) ;
#14035=CARTESIAN_POINT('',(-1.77315669670464,0.70925449161544,0.693233143280018)) ;
#14036=CARTESIAN_POINT('Origin',(-1.75,0.7,0.695)) ;
#14037=CARTESIAN_POINT('Origin',(-1.75,0.7,0.695)) ;
#14038=CARTESIAN_POINT('Origin',(-1.67677669529664,0.876776695296637,0.66125)) ;
#14039=CARTESIAN_POINT('',(-1.68009181793552,0.87346157265775,0.636693536008247)) ;
#14040=CARTESIAN_POINT('',(-1.69993339200128,0.886031186912077,0.659483143280018)) ;
#14041=CARTESIAN_POINT('Origin',(-1.67677669529664,0.876776695296637,0.66125)) ;
#14042=CARTESIAN_POINT('',(-1.67346157265775,0.880091817935524,0.685806463991753)) ;
#14043=CARTESIAN_POINT('Origin',(-1.67677669529664,0.876776695296637,0.66125)) ;
#14044=CARTESIAN_POINT('',(-1.68715097557442,0.897433883049061,0.65172871317105)) ;
#14045=CARTESIAN_POINT('Origin',(-1.67677669529664,0.876776695296637,0.66125)) ;
#14046=CARTESIAN_POINT('Origin',(-1.67677669529664,0.876776695296637,0.66125)) ;
#14047=CARTESIAN_POINT('Origin',(-1.5,0.95,0.6275)) ;
#14048=CARTESIAN_POINT('',(-1.50468829139684,0.95,0.602943536008246)) ;
#14049=CARTESIAN_POINT('',(-1.51037428027778,0.970657187752424,0.61797871317105)) ;
#14050=CARTESIAN_POINT('Origin',(-1.5,0.95,0.6275)) ;
#14051=CARTESIAN_POINT('',(-1.49531170860316,0.95,0.652056463991753)) ;
#14052=CARTESIAN_POINT('Origin',(-1.5,0.95,0.6275)) ;
#14053=CARTESIAN_POINT('Origin',(-1.5,0.95,0.6275)) ;
#14054=CARTESIAN_POINT('Origin',(-1.32322330470336,0.876776695296637,0.59375)) ;
#14055=CARTESIAN_POINT('',(-1.32653842734225,0.880091817935524,0.569193536008247)) ;
#14056=CARTESIAN_POINT('',(-1.31990818206448,0.87346157265775,0.618306463991753)) ;
#14057=CARTESIAN_POINT('Origin',(-1.32322330470336,0.876776695296637,0.59375)) ;
#14058=CARTESIAN_POINT('Origin',(-1.32322330470336,0.876776695296637,0.59375)) ;
#14059=CARTESIAN_POINT('Origin',(-1.28661165235168,0.611611652351681,1.893125)) ;
#14060=CARTESIAN_POINT('',(-1.27315669670464,0.70925449161544,1.91176685671998)) ;
#14061=CARTESIAN_POINT('Origin',(-1.25,0.7,1.91)) ;
#14062=CARTESIAN_POINT('',(-1.34258615076189,0.541636962002279,1.87976551392448)) ;
#14063=CARTESIAN_POINT('',(-1.30976834905632,0.620866143967122,1.89489185671998)) ;
#14064=CARTESIAN_POINT('',(-1.34236685176283,0.540248143222746,1.88409706866696)) ;
#14065=CARTESIAN_POINT('Origin',(-1.32322330470336,0.523223304703363,1.87625)) ;
#14066=CARTESIAN_POINT('Origin',(-1.32322330470336,0.523223304703363,1.87625)) ;
#14067=CARTESIAN_POINT('Origin',(-1.32322330470336,0.523223304703363,1.87625)) ;
#14068=CARTESIAN_POINT('Origin',(-1.25,0.7,1.91)) ;
#14069=CARTESIAN_POINT('Origin',(-1.41161165235168,0.486611652351681,1.859375)) ;
#14070=CARTESIAN_POINT('',(-1.50211870854008,0.474076757531324,1.85359743093369)) ;
#14071=CARTESIAN_POINT('',(-1.42198593262946,0.507268840104105,1.86889628682895)) ;
#14072=CARTESIAN_POINT('Origin',(-1.5,0.45,1.8425)) ;
#14073=CARTESIAN_POINT('Origin',(-1.5,0.45,1.8425)) ;
#14074=CARTESIAN_POINT('Origin',(-1.58838834764832,0.486611652351682,1.825625)) ;
#14075=CARTESIAN_POINT('',(-1.5987626279261,0.465954464599258,1.83514628682895)) ;
#14076=CARTESIAN_POINT('Origin',(-1.67677669529664,0.523223304703363,1.80875)) ;
#14077=CARTESIAN_POINT('Origin',(-1.71338834764832,0.611611652351682,1.791875)) ;
#14078=CARTESIAN_POINT('',(-1.73654504435296,0.602357160736241,1.79364185671998)) ;
#14079=CARTESIAN_POINT('Origin',(-1.75,0.7,1.775)) ;
#14080=CARTESIAN_POINT('Origin',(-1.71338834764832,0.788388347648319,1.758125)) ;
#14081=CARTESIAN_POINT('',(-1.73654504435296,0.797642839263759,1.75635814328002)) ;
#14082=CARTESIAN_POINT('Origin',(-1.67677669529664,0.876776695296637,1.74125)) ;
#14083=CARTESIAN_POINT('Origin',(-1.58838834764832,0.913388347648319,1.724375)) ;
#14084=CARTESIAN_POINT('',(-1.5987626279261,0.934045535400743,1.71485371317105)) ;
#14085=CARTESIAN_POINT('',(-1.50211870854008,0.925923242468676,1.69640256906631)) ;
#14086=CARTESIAN_POINT('Origin',(-1.5,0.95,1.7075)) ;
#14087=CARTESIAN_POINT('Origin',(-1.5,0.95,1.7075)) ;
#14088=CARTESIAN_POINT('Origin',(-1.41161165235168,0.913388347648318,1.690625)) ;
#14089=CARTESIAN_POINT('',(-1.34236685176283,0.859751856777253,1.66590293133304)) ;
#14090=CARTESIAN_POINT('',(-1.42198593262946,0.892731159895895,1.68110371317105)) ;
#14091=CARTESIAN_POINT('',(-1.34258615076189,0.858363037997721,1.67023448607552)) ;
#14092=CARTESIAN_POINT('Origin',(-1.32322330470336,0.876776695296637,1.67375)) ;
#14093=CARTESIAN_POINT('Origin',(-1.32322330470336,0.876776695296637,1.67375)) ;
#14094=CARTESIAN_POINT('Origin',(-1.32322330470336,0.876776695296637,1.67375)) ;
#14095=CARTESIAN_POINT('Origin',(-1.28661165235168,0.788388347648318,1.656875)) ;
#14096=CARTESIAN_POINT('',(-1.27699003264463,0.7,1.64)) ;
#14097=CARTESIAN_POINT('',(-1.30976834905632,0.779133856032878,1.65510814328002)) ;
#14098=CARTESIAN_POINT('Origin',(-1.25,0.7,1.64)) ;
#14099=CARTESIAN_POINT('Origin',(-1.25,0.7,1.64)) ;
#14100=CARTESIAN_POINT('Origin',(-1.28661165235168,0.611611652351681,1.623125)) ;
#14101=CARTESIAN_POINT('',(-1.34258615076189,0.541636962002279,1.60976551392448)) ;
#14102=CARTESIAN_POINT('',(-1.30976834905632,0.620866143967122,1.62489185671998)) ;
#14103=CARTESIAN_POINT('',(-1.34236685176283,0.540248143222746,1.61409706866696)) ;
#14104=CARTESIAN_POINT('Origin',(-1.32322330470336,0.523223304703363,1.60625)) ;
#14105=CARTESIAN_POINT('Origin',(-1.32322330470336,0.523223304703363,1.60625)) ;
#14106=CARTESIAN_POINT('Origin',(-1.32322330470336,0.523223304703363,1.60625)) ;
#14107=CARTESIAN_POINT('Origin',(-1.41161165235168,0.486611652351681,1.589375)) ;
#14108=CARTESIAN_POINT('',(-1.50211870854008,0.474076757531324,1.58359743093369)) ;
#14109=CARTESIAN_POINT('',(-1.42198593262946,0.507268840104105,1.59889628682895)) ;
#14110=CARTESIAN_POINT('Origin',(-1.5,0.45,1.5725)) ;
#14111=CARTESIAN_POINT('Origin',(-1.5,0.45,1.5725)) ;
#14112=CARTESIAN_POINT('Origin',(-1.58838834764832,0.486611652351682,1.555625)) ;
#14113=CARTESIAN_POINT('',(-1.5987626279261,0.465954464599258,1.56514628682895)) ;
#14114=CARTESIAN_POINT('Origin',(-1.67677669529664,0.523223304703363,1.53875)) ;
#14115=CARTESIAN_POINT('Origin',(-1.71338834764832,0.611611652351682,1.521875)) ;
#14116=CARTESIAN_POINT('',(-1.73654504435296,0.602357160736241,1.52364185671998)) ;
#14117=CARTESIAN_POINT('Origin',(-1.75,0.7,1.505)) ;
#14118=CARTESIAN_POINT('Origin',(-1.71338834764832,0.788388347648319,1.488125)) ;
#14119=CARTESIAN_POINT('',(-1.73654504435296,0.797642839263759,1.48635814328002)) ;
#14120=CARTESIAN_POINT('Origin',(-1.67677669529664,0.876776695296637,1.47125)) ;
#14121=CARTESIAN_POINT('Origin',(-1.58838834764832,0.913388347648319,1.454375)) ;
#14122=CARTESIAN_POINT('',(-1.5987626279261,0.934045535400743,1.44485371317105)) ;
#14123=CARTESIAN_POINT('',(-1.50211870854008,0.925923242468676,1.42640256906631)) ;
#14124=CARTESIAN_POINT('Origin',(-1.5,0.95,1.4375)) ;
#14125=CARTESIAN_POINT('Origin',(-1.5,0.95,1.4375)) ;
#14126=CARTESIAN_POINT('Origin',(-1.41161165235168,0.913388347648318,1.420625)) ;
#14127=CARTESIAN_POINT('',(-1.34236685176283,0.859751856777253,1.39590293133304)) ;
#14128=CARTESIAN_POINT('',(-1.42198593262946,0.892731159895895,1.41110371317105)) ;
#14129=CARTESIAN_POINT('',(-1.34258615076189,0.858363037997721,1.40023448607552)) ;
#14130=CARTESIAN_POINT('Origin',(-1.32322330470336,0.876776695296637,1.40375)) ;
#14131=CARTESIAN_POINT('Origin',(-1.32322330470336,0.876776695296637,1.40375)) ;
#14132=CARTESIAN_POINT('Origin',(-1.32322330470336,0.876776695296637,1.40375)) ;
#14133=CARTESIAN_POINT('Origin',(-1.28661165235168,0.788388347648318,1.386875)) ;
#14134=CARTESIAN_POINT('',(-1.27699003264463,0.7,1.37)) ;
#14135=CARTESIAN_POINT('',(-1.30976834905632,0.779133856032878,1.38510814328002)) ;
#14136=CARTESIAN_POINT('Origin',(-1.25,0.7,1.37)) ;
#14137=CARTESIAN_POINT('Origin',(-1.25,0.7,1.37)) ;
#14138=CARTESIAN_POINT('Origin',(-1.28661165235168,0.611611652351681,1.353125)) ;
#14139=CARTESIAN_POINT('',(-1.34258615076189,0.541636962002279,1.33976551392448)) ;
#14140=CARTESIAN_POINT('',(-1.30976834905632,0.620866143967122,1.35489185671998)) ;
#14141=CARTESIAN_POINT('',(-1.34236685176283,0.540248143222746,1.34409706866696)) ;
#14142=CARTESIAN_POINT('Origin',(-1.32322330470336,0.523223304703363,1.33625)) ;
#14143=CARTESIAN_POINT('Origin',(-1.32322330470336,0.523223304703363,1.33625)) ;
#14144=CARTESIAN_POINT('Origin',(-1.32322330470336,0.523223304703363,1.33625)) ;
#14145=CARTESIAN_POINT('Origin',(-1.41161165235168,0.486611652351681,1.319375)) ;
#14146=CARTESIAN_POINT('',(-1.50211870854008,0.474076757531324,1.31359743093369)) ;
#14147=CARTESIAN_POINT('',(-1.42198593262946,0.507268840104105,1.32889628682895)) ;
#14148=CARTESIAN_POINT('Origin',(-1.5,0.45,1.3025)) ;
#14149=CARTESIAN_POINT('Origin',(-1.5,0.45,1.3025)) ;
#14150=CARTESIAN_POINT('Origin',(-1.58838834764832,0.486611652351682,1.285625)) ;
#14151=CARTESIAN_POINT('',(-1.5987626279261,0.465954464599258,1.29514628682895)) ;
#14152=CARTESIAN_POINT('Origin',(-1.67677669529664,0.523223304703363,1.26875)) ;
#14153=CARTESIAN_POINT('Origin',(-1.71338834764832,0.611611652351682,1.251875)) ;
#14154=CARTESIAN_POINT('',(-1.73654504435296,0.602357160736241,1.25364185671998)) ;
#14155=CARTESIAN_POINT('Origin',(-1.75,0.7,1.235)) ;
#14156=CARTESIAN_POINT('Origin',(-1.71338834764832,0.788388347648319,1.218125)) ;
#14157=CARTESIAN_POINT('',(-1.73654504435296,0.797642839263759,1.21635814328002)) ;
#14158=CARTESIAN_POINT('Origin',(-1.67677669529664,0.876776695296637,1.20125)) ;
#14159=CARTESIAN_POINT('Origin',(-1.58838834764832,0.913388347648319,1.184375)) ;
#14160=CARTESIAN_POINT('',(-1.5987626279261,0.934045535400743,1.17485371317105)) ;
#14161=CARTESIAN_POINT('',(-1.50211870854008,0.925923242468676,1.15640256906631)) ;
#14162=CARTESIAN_POINT('Origin',(-1.5,0.95,1.1675)) ;
#14163=CARTESIAN_POINT('Origin',(-1.5,0.95,1.1675)) ;
#14164=CARTESIAN_POINT('Origin',(-1.41161165235168,0.913388347648318,1.150625)) ;
#14165=CARTESIAN_POINT('',(-1.34236685176283,0.859751856777253,1.12590293133304)) ;
#14166=CARTESIAN_POINT('',(-1.42198593262946,0.892731159895895,1.14110371317105)) ;
#14167=CARTESIAN_POINT('',(-1.34258615076189,0.858363037997721,1.13023448607552)) ;
#14168=CARTESIAN_POINT('Origin',(-1.32322330470336,0.876776695296637,1.13375)) ;
#14169=CARTESIAN_POINT('Origin',(-1.32322330470336,0.876776695296637,1.13375)) ;
#14170=CARTESIAN_POINT('Origin',(-1.32322330470336,0.876776695296637,1.13375)) ;
#14171=CARTESIAN_POINT('Origin',(-1.28661165235168,0.788388347648318,1.116875)) ;
#14172=CARTESIAN_POINT('',(-1.27699003264463,0.7,1.1)) ;
#14173=CARTESIAN_POINT('',(-1.30976834905632,0.779133856032878,1.11510814328002)) ;
#14174=CARTESIAN_POINT('Origin',(-1.25,0.7,1.1)) ;
#14175=CARTESIAN_POINT('Origin',(-1.25,0.7,1.1)) ;
#14176=CARTESIAN_POINT('Origin',(-1.28661165235168,0.611611652351681,1.083125)) ;
#14177=CARTESIAN_POINT('',(-1.34258615076189,0.541636962002279,1.06976551392448)) ;
#14178=CARTESIAN_POINT('',(-1.30976834905632,0.620866143967122,1.08489185671998)) ;
#14179=CARTESIAN_POINT('',(-1.34236685176283,0.540248143222746,1.07409706866696)) ;
#14180=CARTESIAN_POINT('Origin',(-1.32322330470336,0.523223304703363,1.06625)) ;
#14181=CARTESIAN_POINT('Origin',(-1.32322330470336,0.523223304703363,1.06625)) ;
#14182=CARTESIAN_POINT('Origin',(-1.32322330470336,0.523223304703363,1.06625)) ;
#14183=CARTESIAN_POINT('Origin',(-1.41161165235168,0.486611652351681,1.049375)) ;
#14184=CARTESIAN_POINT('',(-1.50211870854008,0.474076757531324,1.04359743093369)) ;
#14185=CARTESIAN_POINT('',(-1.42198593262946,0.507268840104105,1.05889628682895)) ;
#14186=CARTESIAN_POINT('Origin',(-1.5,0.45,1.0325)) ;
#14187=CARTESIAN_POINT('Origin',(-1.5,0.45,1.0325)) ;
#14188=CARTESIAN_POINT('Origin',(-1.58838834764832,0.486611652351682,1.015625)) ;
#14189=CARTESIAN_POINT('',(-1.5987626279261,0.465954464599258,1.02514628682895)) ;
#14190=CARTESIAN_POINT('Origin',(-1.67677669529664,0.523223304703363,0.99875)) ;
#14191=CARTESIAN_POINT('Origin',(-1.71338834764832,0.611611652351682,0.981875)) ;
#14192=CARTESIAN_POINT('',(-1.73654504435296,0.602357160736241,0.983641856719982)) ;
#14193=CARTESIAN_POINT('Origin',(-1.75,0.7,0.965)) ;
#14194=CARTESIAN_POINT('Origin',(-1.71338834764832,0.788388347648319,0.948125)) ;
#14195=CARTESIAN_POINT('',(-1.73654504435296,0.797642839263759,0.946358143280018)) ;
#14196=CARTESIAN_POINT('Origin',(-1.67677669529664,0.876776695296637,0.93125)) ;
#14197=CARTESIAN_POINT('Origin',(-1.58838834764832,0.913388347648319,0.914375)) ;
#14198=CARTESIAN_POINT('',(-1.5987626279261,0.934045535400743,0.90485371317105)) ;
#14199=CARTESIAN_POINT('',(-1.50211870854008,0.925923242468676,0.886402569066309)) ;
#14200=CARTESIAN_POINT('Origin',(-1.5,0.95,0.8975)) ;
#14201=CARTESIAN_POINT('Origin',(-1.5,0.95,0.8975)) ;
#14202=CARTESIAN_POINT('Origin',(-1.41161165235168,0.913388347648318,0.880625)) ;
#14203=CARTESIAN_POINT('',(-1.34236685176283,0.859751856777253,0.855902931333038)) ;
#14204=CARTESIAN_POINT('',(-1.42198593262946,0.892731159895895,0.87110371317105)) ;
#14205=CARTESIAN_POINT('',(-1.34258615076189,0.858363037997721,0.860234486075523)) ;
#14206=CARTESIAN_POINT('Origin',(-1.32322330470336,0.876776695296637,0.86375)) ;
#14207=CARTESIAN_POINT('Origin',(-1.32322330470336,0.876776695296637,0.86375)) ;
#14208=CARTESIAN_POINT('Origin',(-1.32322330470336,0.876776695296637,0.86375)) ;
#14209=CARTESIAN_POINT('Origin',(-1.28661165235168,0.788388347648318,0.846875)) ;
#14210=CARTESIAN_POINT('',(-1.27699003264463,0.7,0.83)) ;
#14211=CARTESIAN_POINT('',(-1.30976834905632,0.779133856032878,0.845108143280018)) ;
#14212=CARTESIAN_POINT('Origin',(-1.25,0.7,0.83)) ;
#14213=CARTESIAN_POINT('Origin',(-1.25,0.7,0.83)) ;
#14214=CARTESIAN_POINT('Origin',(-1.28661165235168,0.611611652351681,0.813125)) ;
#14215=CARTESIAN_POINT('',(-1.34258615076189,0.541636962002279,0.799765513924477)) ;
#14216=CARTESIAN_POINT('',(-1.30976834905632,0.620866143967122,0.814891856719982)) ;
#14217=CARTESIAN_POINT('',(-1.34236685176283,0.540248143222747,0.804097068666963)) ;
#14218=CARTESIAN_POINT('Origin',(-1.32322330470336,0.523223304703363,0.79625)) ;
#14219=CARTESIAN_POINT('Origin',(-1.32322330470336,0.523223304703363,0.79625)) ;
#14220=CARTESIAN_POINT('Origin',(-1.32322330470336,0.523223304703363,0.79625)) ;
#14221=CARTESIAN_POINT('Origin',(-1.41161165235168,0.486611652351682,0.779375)) ;
#14222=CARTESIAN_POINT('',(-1.50211870854008,0.474076757531324,0.773597430933691)) ;
#14223=CARTESIAN_POINT('',(-1.42198593262946,0.507268840104105,0.78889628682895)) ;
#14224=CARTESIAN_POINT('Origin',(-1.5,0.45,0.7625)) ;
#14225=CARTESIAN_POINT('Origin',(-1.5,0.45,0.7625)) ;
#14226=CARTESIAN_POINT('Origin',(-1.58838834764832,0.486611652351682,0.745625)) ;
#14227=CARTESIAN_POINT('',(-1.5987626279261,0.465954464599258,0.75514628682895)) ;
#14228=CARTESIAN_POINT('Origin',(-1.67677669529664,0.523223304703363,0.72875)) ;
#14229=CARTESIAN_POINT('Origin',(-1.71338834764832,0.611611652351682,0.711875)) ;
#14230=CARTESIAN_POINT('',(-1.73654504435296,0.602357160736241,0.713641856719982)) ;
#14231=CARTESIAN_POINT('Origin',(-1.75,0.7,0.695)) ;
#14232=CARTESIAN_POINT('Origin',(-1.71338834764832,0.788388347648318,0.678125)) ;
#14233=CARTESIAN_POINT('',(-1.73654504435296,0.797642839263759,0.676358143280018)) ;
#14234=CARTESIAN_POINT('Origin',(-1.67677669529664,0.876776695296637,0.66125)) ;
#14235=CARTESIAN_POINT('Origin',(-1.58838834764832,0.913388347648318,0.644375)) ;
#14236=CARTESIAN_POINT('',(-1.5987626279261,0.934045535400742,0.63485371317105)) ;
#14237=CARTESIAN_POINT('',(-1.50211870854008,0.925923242468676,0.616402569066309)) ;
#14238=CARTESIAN_POINT('Origin',(-1.5,0.95,0.6275)) ;
#14239=CARTESIAN_POINT('Origin',(-1.5,0.95,0.6275)) ;
#14240=CARTESIAN_POINT('Origin',(-1.41161165235168,0.913388347648318,0.610625)) ;
#14241=CARTESIAN_POINT('',(-1.34236685176283,0.859751856777253,0.585902931333038)) ;
#14242=CARTESIAN_POINT('',(-1.42198593262946,0.892731159895895,0.60110371317105)) ;
#14243=CARTESIAN_POINT('',(-1.34258615076189,0.858363037997721,0.590234486075523)) ;
#14244=CARTESIAN_POINT('Origin',(-1.32322330470336,0.876776695296637,0.59375)) ;
#14245=CARTESIAN_POINT('Origin',(-1.32322330470336,0.876776695296637,0.59375)) ;
#14246=CARTESIAN_POINT('Origin',(-1.32322330470336,0.876776695296637,0.59375)) ;
#14247=CARTESIAN_POINT('Origin',(-1.28661165235168,0.788388347648318,0.576875)) ;
#14248=CARTESIAN_POINT('',(-1.27315669670464,0.690745508384559,0.558233143280018)) ;
#14249=CARTESIAN_POINT('',(-1.30976834905632,0.779133856032878,0.575108143280018)) ;
#14250=CARTESIAN_POINT('Origin',(-1.25,0.7,0.56)) ;
#14251=CARTESIAN_POINT('Origin',(-1.25,0.7,0.56)) ;
#15421=UNCERTAINTY_MEASURE_WITH_UNIT(LENGTH_MEASURE(0.001),#15485,
'DISTANCE_ACCURACY_VALUE',
'Maximum model space distance between geometric entities at asserted c
onnectivities') ;
#15441=UNCERTAINTY_MEASURE_WITH_UNIT(LENGTH_MEASURE(0.001),#15485,
'DISTANCE_ACCURACY_VALUE',
'Maximum model space distance between geometric entities at asserted c
onnectivities') ;
#15464=(
GEOMETRIC_REPRESENTATION_CONTEXT(3)
GLOBAL_UNCERTAINTY_ASSIGNED_CONTEXT((#15421))
GLOBAL_UNIT_ASSIGNED_CONTEXT((#15485,#15487,#15488))
REPRESENTATION_CONTEXT('','3D')
) ;
#15484=(
GEOMETRIC_REPRESENTATION_CONTEXT(3)
GLOBAL_UNCERTAINTY_ASSIGNED_CONTEXT((#15441))
GLOBAL_UNIT_ASSIGNED_CONTEXT((#15485,#15487,#15488))
REPRESENTATION_CONTEXT('','3D')
) ;
#15485=(
LENGTH_UNIT()
NAMED_UNIT(*)
SI_UNIT(.CENTI.,.METRE.)
) ;
#15487=(
NAMED_UNIT(*)
PLANE_ANGLE_UNIT()
SI_UNIT($,.RADIAN.)
) ;
#15488=(
NAMED_UNIT(*)
SI_UNIT($,.STERADIAN.)
SOLID_ANGLE_UNIT()
) ;
#15511=SHAPE_DEFINITION_REPRESENTATION(#15568,#15640) ;
#15568=PRODUCT_DEFINITION_SHAPE('',$,#15683) ;
#15640=SHAPE_REPRESENTATION('',(#9044),#15464) ;
#15660=PRODUCT_DEFINITION_CONTEXT('part definition',#15788,'design') ;
#15683=PRODUCT_DEFINITION('TRIP_LEVER_RETURN_SPRING',
'TRIP_LEVER_RETURN_SPRING',#15725,#15660) ;
#15725=PRODUCT_DEFINITION_FORMATION('',$,#15812) ;
#15788=APPLICATION_CONTEXT(
'Core Data for Automotive Mechanical Design Process') ;
#15789=PRODUCT_CONTEXT('part definition',#15788,'mechanical') ;
#15812=PRODUCT('TRIP_LEVER_RETURN_SPRING','TRIP_LEVER_RETURN_SPRING',$,(#15789)) ;
#15832=PRESENTATION_STYLE_ASSIGNMENT((#15844)) ;
#15844=SURFACE_STYLE_USAGE(.BOTH.,#15856) ;
#15856=SURFACE_SIDE_STYLE('',(#15868)) ;
#15868=SURFACE_STYLE_FILL_AREA(#15880) ;
#15880=FILL_AREA_STYLE('Steel - Satin',(#15892)) ;
#15892=FILL_AREA_STYLE_COLOUR('Steel - Satin',#15904) ;
#15904=COLOUR_RGB('Steel - Satin', 0.72549020, 0.75294118, 0.79215686) ;
ENDSEC;
END-ISO-10303-21;
